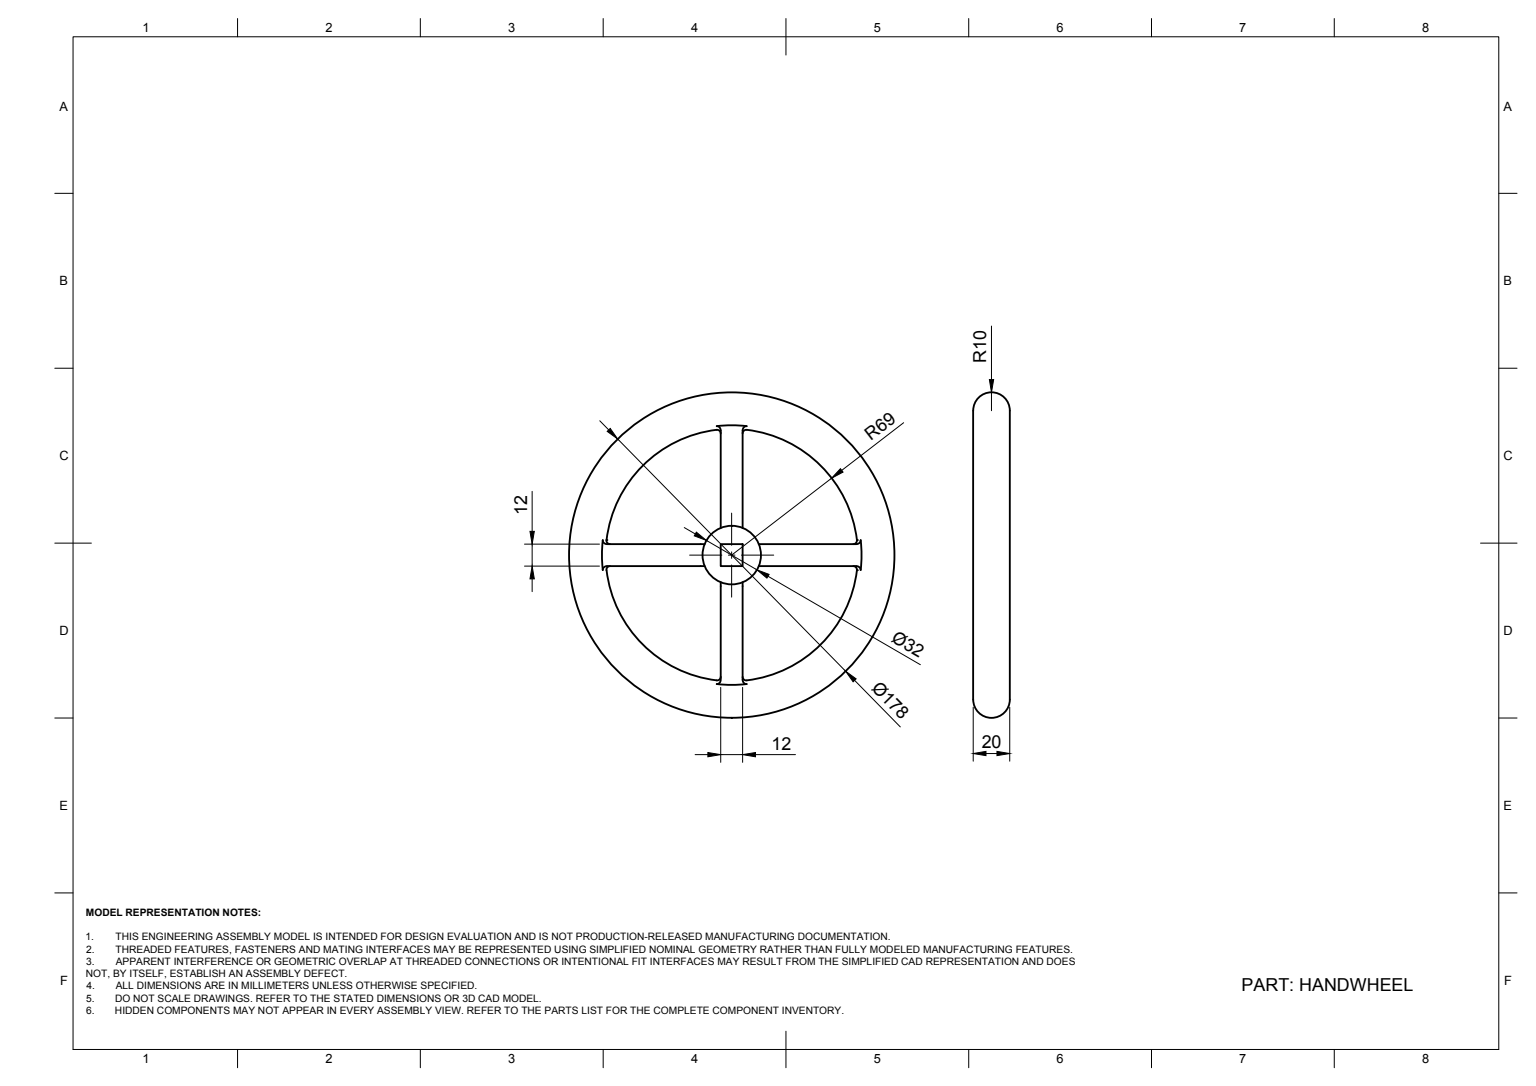
ISO-10303-21;
HEADER;
/* Generated by software containing ST-Developer
 * from STEP Tools, Inc. (www.steptools.com) 
 */

FILE_DESCRIPTION(
/* description */ (''),
/* implementation_level */ '2;1');

FILE_NAME(
/* name */ 'HANDWHEEL.step',
/* time_stamp */ '2026-10-04T02:10:06-07:00',
/* author */ (''),
/* organization */ (''),
/* preprocessor_version */ 'ST-DEVELOPER v20.2',
/* originating_system */ 'Autodesk Translation Framework v15.15.0.0',
/* authorisation */ '');

FILE_SCHEMA (('AUTOMOTIVE_DESIGN { 1 0 10303 214 3 1 1 }'));
ENDSEC;

DATA;
#10=MECHANICAL_DESIGN_GEOMETRIC_PRESENTATION_REPRESENTATION('',(#149),#9668);
#67=(
BOUNDED_SURFACE()
B_SPLINE_SURFACE(3,2,((#8974,#8975,#8976),(#8977,#8978,#8979),(#8980,#8981,
#8982),(#8983,#8984,#8985),(#8986,#8987,#8988),(#8989,#8990,#8991),(#8992,
#8993,#8994),(#8995,#8996,#8997),(#8998,#8999,#9000),(#9001,#9002,#9003),
(#9004,#9005,#9006),(#9007,#9008,#9009),(#9010,#9011,#9012),(#9013,#9014,
#9015),(#9016,#9017,#9018),(#9019,#9020,#9021),(#9022,#9023,#9024),(#9025,
#9026,#9027)),.UNSPECIFIED.,.F.,.F.,.F.)
B_SPLINE_SURFACE_WITH_KNOTS((4,1,1,1,1,1,1,1,1,1,1,1,1,1,1,4),(3,3),(0.0314788030428868,
0.0324522874563819,0.0334257718698771,0.0353727406968673,0.0363462251103625,
0.0373197095238576,0.0382931939373528,0.0392666783508479,0.0402401627643431,
0.0412136471778382,0.0421871315913334,0.0431606160048285,0.0441341004183236,
0.0451075848318188,0.0460810692453139,0.0470545536588091),(0.,1.),
 .UNSPECIFIED.)
GEOMETRIC_REPRESENTATION_ITEM()
RATIONAL_B_SPLINE_SURFACE(((1.,0.673965297618148,1.),(1.,0.673166296515258,
1.),(1.,0.671622878424884,1.),(1.,0.668872043360916,1.),(1.,0.6666737415125,
1.),(1.,0.665066367000124,1.),(1.,0.664191179384959,1.),(1.,0.663664801981856,
1.),(1.,0.663490402453091,1.),(1.,0.663673371681184,1.),(1.,0.664201607885415,
1.),(1.,0.66506767873011,1.),(1.,0.666279408316226,1.),(1.,0.667792932640577,
1.),(1.,0.669583017900756,1.),(1.,0.671633975311695,1.),(1.,0.673174922786531,
1.),(1.,0.673980190168732,1.)))
REPRESENTATION_ITEM('')
SURFACE()
);
#68=(
BOUNDED_SURFACE()
B_SPLINE_SURFACE(3,2,((#9028,#9029,#9030),(#9031,#9032,#9033),(#9034,#9035,
#9036),(#9037,#9038,#9039),(#9040,#9041,#9042),(#9043,#9044,#9045),(#9046,
#9047,#9048),(#9049,#9050,#9051),(#9052,#9053,#9054),(#9055,#9056,#9057),
(#9058,#9059,#9060),(#9061,#9062,#9063),(#9064,#9065,#9066),(#9067,#9068,
#9069),(#9070,#9071,#9072),(#9073,#9074,#9075),(#9076,#9077,#9078),(#9079,
#9080,#9081)),.UNSPECIFIED.,.F.,.F.,.F.)
B_SPLINE_SURFACE_WITH_KNOTS((4,1,1,1,1,1,1,1,1,1,1,1,1,1,1,4),(3,3),(0.0306904631349172,
0.0316643361466102,0.0326382091583032,0.0336120821699963,0.0345859551816893,
0.0355598281933823,0.0365337012050753,0.0375075742167683,0.0384814472284614,
0.0394553202401544,0.0404291932518474,0.0414030662635404,0.0423769392752334,
0.0433508122869265,0.0443246852986195,0.0462724313220055),(0.,1.),
 .UNSPECIFIED.)
GEOMETRIC_REPRESENTATION_ITEM()
RATIONAL_B_SPLINE_SURFACE(((1.,0.673964349039136,1.),(1.,0.673168502978567,
1.),(1.,0.671643925861953,1.),(1.,0.669562296886318,1.),(1.,0.667767007356651,
1.),(1.,0.666266776870979,1.),(1.,0.665071978074277,1.),(1.,0.664194007330874,
1.),(1.,0.663665542131989,1.),(1.,0.663490103902602,1.),(1.,0.663673710164509,
1.),(1.,0.664205908065376,1.),(1.,0.665074561266886,1.),(1.,0.666270920547672,
1.),(1.,0.667799410011383,1.),(1.,0.670197938500333,1.),(1.,0.672375755500364,
1.),(1.,0.673978916833767,1.)))
REPRESENTATION_ITEM('')
SURFACE()
);
#69=(
BOUNDED_SURFACE()
B_SPLINE_SURFACE(3,2,((#9082,#9083,#9084),(#9085,#9086,#9087),(#9088,#9089,
#9090),(#9091,#9092,#9093),(#9094,#9095,#9096),(#9097,#9098,#9099),(#9100,
#9101,#9102),(#9103,#9104,#9105),(#9106,#9107,#9108),(#9109,#9110,#9111),
(#9112,#9113,#9114),(#9115,#9116,#9117),(#9118,#9119,#9120),(#9121,#9122,
#9123),(#9124,#9125,#9126),(#9127,#9128,#9129),(#9130,#9131,#9132),(#9133,
#9134,#9135)),.UNSPECIFIED.,.F.,.F.,.F.)
B_SPLINE_SURFACE_WITH_KNOTS((4,1,1,1,1,1,1,1,1,1,1,1,1,1,1,4),(3,3),(0.0305897871911959,
0.0315636944986189,0.0325376018060419,0.0335115091134649,0.0344854164208879,
0.0354593237283109,0.0364332310357338,0.0374071383431568,0.0383810456505798,
0.0393549529580028,0.0403288602654258,0.0413027675728487,0.0422766748802717,
0.0432505821876947,0.0442244894951177,0.0461723041099637),(0.,1.),
 .UNSPECIFIED.)
GEOMETRIC_REPRESENTATION_ITEM()
RATIONAL_B_SPLINE_SURFACE(((1.,0.673964296834234,1.),(1.,0.673168609933157,
1.),(1.,0.671645019887839,1.),(1.,0.669565127304379,1.),(1.,0.667766560497273,
1.),(1.,0.666266474426915,1.),(1.,0.66507215658795,1.),(1.,0.664195156886529,
1.),(1.,0.663665573830476,1.),(1.,0.663490167959275,1.),(1.,0.663673406028792,
1.),(1.,0.664206149646574,1.),(1.,0.665075135400244,1.),(1.,0.666270395103817,
1.),(1.,0.667798233506142,1.),(1.,0.670199686629813,1.),(1.,0.672377030394903,
1.),(1.,0.673978715902987,1.)))
REPRESENTATION_ITEM('')
SURFACE()
);
#70=(
BOUNDED_SURFACE()
B_SPLINE_SURFACE(3,2,((#9136,#9137,#9138),(#9139,#9140,#9141),(#9142,#9143,
#9144),(#9145,#9146,#9147),(#9148,#9149,#9150),(#9151,#9152,#9153),(#9154,
#9155,#9156),(#9157,#9158,#9159),(#9160,#9161,#9162),(#9163,#9164,#9165),
(#9166,#9167,#9168),(#9169,#9170,#9171),(#9172,#9173,#9174),(#9175,#9176,
#9177),(#9178,#9179,#9180),(#9181,#9182,#9183),(#9184,#9185,#9186),(#9187,
#9188,#9189)),.UNSPECIFIED.,.F.,.F.,.F.)
B_SPLINE_SURFACE_WITH_KNOTS((4,1,1,1,1,1,1,1,1,1,1,1,1,1,1,4),(3,3),(0.0315789108977846,
0.0325523529389518,0.0335257949801189,0.0354726790624532,0.0364461211036204,
0.0374195631447876,0.0383930051859547,0.0393664472271219,0.040339889268289,
0.0413133313094562,0.0422867733506233,0.0432602153917905,0.0442336574329576,
0.0452070994741248,0.046180541515292,0.0471539835564591),(0.,1.),
 .UNSPECIFIED.)
GEOMETRIC_REPRESENTATION_ITEM()
RATIONAL_B_SPLINE_SURFACE(((1.,0.673965492863365,1.),(1.,0.673165826863236,
1.),(1.,0.671620469526443,1.),(1.,0.668874652098692,1.),(1.,0.666674941728974,
1.),(1.,0.665065162761098,1.),(1.,0.664191461531519,1.),(1.,0.663664604196809,
1.),(1.,0.663490522562251,1.),(1.,0.663673087023803,1.),(1.,0.664200791428412,
1.),(1.,0.665067176842279,1.),(1.,0.666279817333014,1.),(1.,0.667791010794828,
1.),(1.,0.669580698382089,1.),(1.,0.671631849583161,1.),(1.,0.673175667819509,
1.),(1.,0.673979886421463,1.)))
REPRESENTATION_ITEM('')
SURFACE()
);
#71=(
BOUNDED_SURFACE()
B_SPLINE_SURFACE(3,2,((#9190,#9191,#9192),(#9193,#9194,#9195),(#9196,#9197,
#9198),(#9199,#9200,#9201),(#9202,#9203,#9204),(#9205,#9206,#9207),(#9208,
#9209,#9210),(#9211,#9212,#9213),(#9214,#9215,#9216),(#9217,#9218,#9219),
(#9220,#9221,#9222),(#9223,#9224,#9225),(#9226,#9227,#9228),(#9229,#9230,
#9231),(#9232,#9233,#9234),(#9235,#9236,#9237)),.UNSPECIFIED.,.F.,.F.,.F.)
B_SPLINE_SURFACE_WITH_KNOTS((4,1,1,1,1,1,1,1,1,1,1,1,1,4),(3,3),(0.03215789731342,
0.0331313751868945,0.034104853060369,0.0350783309338435,0.0360518088073179,
0.0370252866807924,0.0379987645542669,0.0389722424277414,0.0399457203012159,
0.0418926760481649,0.0438396317951138,0.0457865875420628,0.0467600654155373,
0.0477335432890118),(-8.08454907084105E-6,1.),.UNSPECIFIED.)
GEOMETRIC_REPRESENTATION_ITEM()
RATIONAL_B_SPLINE_SURFACE(((1.00000527170182,0.673964387359616,1.),(1.00000528471687,
0.673159453411099,1.),(1.00000530961685,0.671619480347489,1.),(1.00000534275063,
0.669570276226346,1.),(1.00000537166522,0.66778201413489,1.),(1.00000539609675,
0.666271012581043,1.),(1.00000541568478,0.665059564372101,1.),(1.00000542974255,
0.664190142086893,1.),(1.000005438313,0.663660090710924,1.),(1.00000544199604,
0.663432308407853,1.),(1.00000543253772,0.664017270646154,1.),(1.00000539844928,
0.666125517336438,1.),(1.00000535391695,0.668879680311451,1.),(1.00000530941503,
0.671631962440139,1.),(1.00000528444356,0.673176357213759,1.),(1.00000527151599,
0.673975880021096,1.)))
REPRESENTATION_ITEM('')
SURFACE()
);
#72=(
BOUNDED_SURFACE()
B_SPLINE_SURFACE(3,2,((#9238,#9239,#9240),(#9241,#9242,#9243),(#9244,#9245,
#9246),(#9247,#9248,#9249),(#9250,#9251,#9252),(#9253,#9254,#9255),(#9256,
#9257,#9258),(#9259,#9260,#9261),(#9262,#9263,#9264),(#9265,#9266,#9267),
(#9268,#9269,#9270),(#9271,#9272,#9273),(#9274,#9275,#9276),(#9277,#9278,
#9279),(#9280,#9281,#9282),(#9283,#9284,#9285)),.UNSPECIFIED.,.F.,.F.,.F.)
B_SPLINE_SURFACE_WITH_KNOTS((4,1,1,1,1,1,1,1,1,1,1,1,1,4),(3,3),(0.0300049518513901,
0.031953018177045,0.0329270513398724,0.0339010845026998,0.0348751176655272,
0.0358491508283546,0.036823183991182,0.0377972171540094,0.0387712503168368,
0.0397452834796642,0.041693349805319,0.0426673829681464,0.0436414161309738,
0.0455894824566286),(0.,1.),.UNSPECIFIED.)
GEOMETRIC_REPRESENTATION_ITEM()
RATIONAL_B_SPLINE_SURFACE(((1.,0.673964297815332,1.),(1.,0.672372618458235,
1.),(1.,0.670191181394266,1.),(1.,0.667767841290405,1.),(1.,0.666265347639804,
1.),(1.,0.665072121147338,1.),(1.,0.664201207028703,1.),(1.,0.663666605647771,
1.),(1.,0.663490715236844,1.),(1.,0.663670119784287,1.),(1.,0.664385152559804,
1.),(1.,0.665767066134064,1.),(1.,0.66778345083312,1.),(1.,0.670206332337341,
1.),(1.,0.672382580991143,1.),(1.,0.673977852527306,1.)))
REPRESENTATION_ITEM('')
SURFACE()
);
#73=(
BOUNDED_SURFACE()
B_SPLINE_SURFACE(3,2,((#9286,#9287,#9288),(#9289,#9290,#9291),(#9292,#9293,
#9294),(#9295,#9296,#9297),(#9298,#9299,#9300),(#9301,#9302,#9303),(#9304,
#9305,#9306),(#9307,#9308,#9309),(#9310,#9311,#9312),(#9313,#9314,#9315),
(#9316,#9317,#9318),(#9319,#9320,#9321),(#9322,#9323,#9324),(#9325,#9326,
#9327),(#9328,#9329,#9330),(#9331,#9332,#9333),(#9334,#9335,#9336),(#9337,
#9338,#9339),(#9340,#9341,#9342)),.UNSPECIFIED.,.F.,.F.,.F.)
B_SPLINE_SURFACE_WITH_KNOTS((4,1,1,1,1,1,1,1,1,1,1,1,1,1,1,1,4),(3,3),(0.0317649381765832,
0.0327383392942574,0.0337117404119316,0.0346851415296058,0.03565854264728,
0.0366319437649542,0.0376053448826284,0.0385787460003026,0.0395521471179768,
0.040525548235651,0.0414989493533253,0.0424723504709995,0.0434457515886737,
0.0444191527063479,0.0453925538240221,0.0463659549416963,0.0473393560593705),
(0.,1.),.UNSPECIFIED.)
GEOMETRIC_REPRESENTATION_ITEM()
RATIONAL_B_SPLINE_SURFACE(((1.,0.673965909365134,1.),(1.,0.673164818236142,
1.),(1.,0.671618061862569,1.),(1.,0.669564320284071,1.),(1.,0.66777759511695,
1.),(1.,0.666273471258361,1.),(1.,0.665063410818969,1.),(1.,0.664191967652661,
1.),(1.,0.663664156821065,1.),(1.,0.663490769293391,1.),(1.,0.663672536496092,
1.),(1.,0.664199292987571,1.),(1.,0.665067031441957,1.),(1.,0.666280071948857,
1.),(1.,0.66778774864528,1.),(1.,0.669576760671401,1.),(1.,0.671629936935393,
1.),(1.,0.673176919539912,1.),(1.,0.673979374441674,1.)))
REPRESENTATION_ITEM('')
SURFACE()
);
#74=(
BOUNDED_SURFACE()
B_SPLINE_SURFACE(3,2,((#9343,#9344,#9345),(#9346,#9347,#9348),(#9349,#9350,
#9351),(#9352,#9353,#9354),(#9355,#9356,#9357),(#9358,#9359,#9360),(#9361,
#9362,#9363),(#9364,#9365,#9366),(#9367,#9368,#9369),(#9370,#9371,#9372),
(#9373,#9374,#9375),(#9376,#9377,#9378),(#9379,#9380,#9381),(#9382,#9383,
#9384),(#9385,#9386,#9387),(#9388,#9389,#9390),(#9391,#9392,#9393)),
 .UNSPECIFIED.,.F.,.F.,.F.)
B_SPLINE_SURFACE_WITH_KNOTS((4,1,1,1,1,1,1,1,1,1,1,1,1,1,4),(3,3),(0.0304023584176636,
0.0313763197495467,0.0323502810814299,0.0333242424133131,0.0342982037451962,
0.0352721650770794,0.0362461264089626,0.0372200877408457,0.0381940490727289,
0.0391680104046121,0.0401419717364953,0.0420898944002616,0.0430638557321448,
0.0440378170640279,0.0459857397277943),(0.,1.),.UNSPECIFIED.)
GEOMETRIC_REPRESENTATION_ITEM()
RATIONAL_B_SPLINE_SURFACE(((1.,0.673964240667089,1.),(1.,0.673168704865034,
1.),(1.,0.671646043506943,1.),(1.,0.669571927360062,1.),(1.,0.667765968900773,
1.),(1.,0.666266091842261,1.),(1.,0.665072243840693,1.),(1.,0.664197515743925,
1.),(1.,0.663665655019745,1.),(1.,0.663490373557035,1.),(1.,0.663672476132646,
1.),(1.,0.664385168150455,1.),(1.,0.665762507320331,1.),(1.,0.667794613454947,
1.),(1.,0.670202685638588,1.),(1.,0.672379152055614,1.),(1.,0.6739783830491,
1.)))
REPRESENTATION_ITEM('')
SURFACE()
);
#127=SHAPE_REPRESENTATION_RELATIONSHIP('SRR','None',#9720,#138);
#138=ADVANCED_BREP_SHAPE_REPRESENTATION('',(#160),#9665);
#149=STYLED_ITEM('',(#9775),#160);
#160=MANIFOLD_SOLID_BREP('Body1',#3889);
#260=FACE_BOUND('',#1262,.T.);
#261=FACE_BOUND('',#1263,.T.);
#262=FACE_BOUND('',#1264,.T.);
#263=FACE_BOUND('',#1266,.T.);
#264=FACE_BOUND('',#1268,.T.);
#332=PLANE('',#4327);
#333=PLANE('',#4328);
#334=PLANE('',#4329);
#335=PLANE('',#4332);
#336=PLANE('',#4336);
#337=PLANE('',#4339);
#338=PLANE('',#4343);
#339=PLANE('',#4346);
#340=PLANE('',#4349);
#341=PLANE('',#4350);
#342=PLANE('',#4351);
#343=PLANE('',#4352);
#344=PLANE('',#4353);
#345=PLANE('',#4354);
#346=PLANE('',#4363);
#347=PLANE('',#4365);
#348=PLANE('',#4380);
#349=PLANE('',#4381);
#350=PLANE('',#4382);
#351=PLANE('',#4383);
#352=PLANE('',#4384);
#353=PLANE('',#4385);
#504=LINE('',#7172,#695);
#505=LINE('',#7263,#696);
#506=LINE('',#7276,#697);
#507=LINE('',#7290,#698);
#508=LINE('',#7384,#699);
#509=LINE('',#7397,#700);
#510=LINE('',#7440,#701);
#511=LINE('',#7444,#702);
#512=LINE('',#7477,#703);
#513=LINE('',#7481,#704);
#514=LINE('',#7512,#705);
#515=LINE('',#7516,#706);
#516=LINE('',#7578,#707);
#517=LINE('',#7582,#708);
#518=LINE('',#7701,#709);
#519=LINE('',#7714,#710);
#520=LINE('',#7728,#711);
#521=LINE('',#7823,#712);
#522=LINE('',#7932,#713);
#523=LINE('',#8044,#714);
#524=LINE('',#8149,#715);
#525=LINE('',#8162,#716);
#526=LINE('',#8176,#717);
#527=LINE('',#8274,#718);
#528=LINE('',#8925,#719);
#529=LINE('',#8930,#720);
#530=LINE('',#8943,#721);
#531=LINE('',#8945,#722);
#532=LINE('',#8947,#723);
#533=LINE('',#8948,#724);
#534=LINE('',#8952,#725);
#535=LINE('',#8954,#726);
#536=LINE('',#8956,#727);
#537=LINE('',#8957,#728);
#538=LINE('',#8959,#729);
#539=LINE('',#8960,#730);
#540=LINE('',#8962,#731);
#541=LINE('',#8964,#732);
#695=VECTOR('',#5230,51.1691161062453);
#696=VECTOR('',#5231,51.1691161062453);
#697=VECTOR('',#5232,16.);
#698=VECTOR('',#5235,51.1691161062453);
#699=VECTOR('',#5236,51.1691161062453);
#700=VECTOR('',#5237,16.);
#701=VECTOR('',#5246,51.1691161062453);
#702=VECTOR('',#5249,51.1691161062452);
#703=VECTOR('',#5256,51.1691161062453);
#704=VECTOR('',#5259,51.1691161062453);
#705=VECTOR('',#5264,51.1691161062453);
#706=VECTOR('',#5267,51.1691161062453);
#707=VECTOR('',#5280,51.1691161062453);
#708=VECTOR('',#5283,51.1691161062453);
#709=VECTOR('',#5288,51.1691161062453);
#710=VECTOR('',#5289,16.);
#711=VECTOR('',#5292,51.1691161062453);
#712=VECTOR('',#5293,16.);
#713=VECTOR('',#5296,16.);
#714=VECTOR('',#5299,16.);
#715=VECTOR('',#5302,51.1691161062453);
#716=VECTOR('',#5303,16.);
#717=VECTOR('',#5306,51.1691161062453);
#718=VECTOR('',#5307,16.);
#719=VECTOR('',#5336,16.);
#720=VECTOR('',#5341,16.);
#721=VECTOR('',#5362,12.);
#722=VECTOR('',#5363,12.);
#723=VECTOR('',#5364,12.);
#724=VECTOR('',#5365,12.);
#725=VECTOR('',#5368,12.);
#726=VECTOR('',#5369,12.);
#727=VECTOR('',#5370,12.);
#728=VECTOR('',#5371,12.);
#729=VECTOR('',#5374,20.);
#730=VECTOR('',#5375,20.);
#731=VECTOR('',#5378,20.);
#732=VECTOR('',#5381,20.);
#807=CYLINDRICAL_SURFACE('',#4367,16.);
#956=FACE_OUTER_BOUND('',#1244,.T.);
#957=FACE_OUTER_BOUND('',#1245,.T.);
#958=FACE_OUTER_BOUND('',#1246,.T.);
#959=FACE_OUTER_BOUND('',#1247,.T.);
#960=FACE_OUTER_BOUND('',#1248,.T.);
#961=FACE_OUTER_BOUND('',#1249,.T.);
#962=FACE_OUTER_BOUND('',#1250,.T.);
#963=FACE_OUTER_BOUND('',#1251,.T.);
#964=FACE_OUTER_BOUND('',#1252,.T.);
#965=FACE_OUTER_BOUND('',#1253,.T.);
#966=FACE_OUTER_BOUND('',#1254,.T.);
#967=FACE_OUTER_BOUND('',#1255,.T.);
#968=FACE_OUTER_BOUND('',#1256,.T.);
#969=FACE_OUTER_BOUND('',#1257,.T.);
#970=FACE_OUTER_BOUND('',#1258,.T.);
#971=FACE_OUTER_BOUND('',#1259,.T.);
#972=FACE_OUTER_BOUND('',#1260,.T.);
#973=FACE_OUTER_BOUND('',#1261,.T.);
#974=FACE_OUTER_BOUND('',#1265,.T.);
#975=FACE_OUTER_BOUND('',#1267,.T.);
#976=FACE_OUTER_BOUND('',#1269,.T.);
#977=FACE_OUTER_BOUND('',#1270,.T.);
#978=FACE_OUTER_BOUND('',#1271,.T.);
#979=FACE_OUTER_BOUND('',#1272,.T.);
#980=FACE_OUTER_BOUND('',#1273,.T.);
#981=FACE_OUTER_BOUND('',#1274,.T.);
#982=FACE_OUTER_BOUND('',#1275,.T.);
#983=FACE_OUTER_BOUND('',#1276,.T.);
#984=FACE_OUTER_BOUND('',#1277,.T.);
#985=FACE_OUTER_BOUND('',#1278,.T.);
#986=FACE_OUTER_BOUND('',#1279,.T.);
#987=FACE_OUTER_BOUND('',#1280,.T.);
#988=FACE_OUTER_BOUND('',#1281,.T.);
#989=FACE_OUTER_BOUND('',#1282,.T.);
#990=FACE_OUTER_BOUND('',#1283,.T.);
#991=FACE_OUTER_BOUND('',#1284,.T.);
#992=FACE_OUTER_BOUND('',#1285,.T.);
#993=FACE_OUTER_BOUND('',#1286,.T.);
#994=FACE_OUTER_BOUND('',#1287,.T.);
#995=FACE_OUTER_BOUND('',#1288,.T.);
#1244=EDGE_LOOP('',(#3221,#3222,#3223,#3224,#3225,#3226));
#1245=EDGE_LOOP('',(#3227,#3228,#3229,#3230,#3231,#3232));
#1246=EDGE_LOOP('',(#3233,#3234,#3235,#3236,#3237,#3238));
#1247=EDGE_LOOP('',(#3239,#3240,#3241,#3242,#3243,#3244,#3245));
#1248=EDGE_LOOP('',(#3246,#3247,#3248,#3249,#3250,#3251));
#1249=EDGE_LOOP('',(#3252,#3253,#3254,#3255,#3256,#3257,#3258));
#1250=EDGE_LOOP('',(#3259,#3260,#3261,#3262,#3263,#3264));
#1251=EDGE_LOOP('',(#3265,#3266,#3267,#3268,#3269,#3270));
#1252=EDGE_LOOP('',(#3271,#3272,#3273,#3274,#3275,#3276));
#1253=EDGE_LOOP('',(#3277,#3278,#3279,#3280,#3281,#3282));
#1254=EDGE_LOOP('',(#3283,#3284,#3285,#3286,#3287,#3288));
#1255=EDGE_LOOP('',(#3289,#3290,#3291,#3292,#3293,#3294));
#1256=EDGE_LOOP('',(#3295,#3296,#3297,#3298,#3299,#3300));
#1257=EDGE_LOOP('',(#3301,#3302,#3303,#3304,#3305,#3306));
#1258=EDGE_LOOP('',(#3307,#3308,#3309,#3310,#3311,#3312,#3313,#3314,#3315,
#3316,#3317,#3318,#3319,#3320,#3321,#3322,#3323,#3324,#3325,#3326,#3327,
#3328,#3329,#3330,#3331,#3332,#3333,#3334,#3335,#3336,#3337,#3338,#3339,
#3340,#3341,#3342));
#1259=EDGE_LOOP('',(#3343,#3344,#3345,#3346,#3347,#3348));
#1260=EDGE_LOOP('',(#3349,#3350,#3351,#3352,#3353,#3354));
#1261=EDGE_LOOP('',(#3355,#3356,#3357,#3358,#3359,#3360,#3361,#3362,#3363,
#3364,#3365,#3366));
#1262=EDGE_LOOP('',(#3367,#3368,#3369,#3370));
#1263=EDGE_LOOP('',(#3371,#3372,#3373,#3374));
#1264=EDGE_LOOP('',(#3375,#3376,#3377,#3378));
#1265=EDGE_LOOP('',(#3379));
#1266=EDGE_LOOP('',(#3380,#3381,#3382,#3383));
#1267=EDGE_LOOP('',(#3384));
#1268=EDGE_LOOP('',(#3385,#3386,#3387,#3388));
#1269=EDGE_LOOP('',(#3389,#3390,#3391,#3392));
#1270=EDGE_LOOP('',(#3393,#3394,#3395,#3396));
#1271=EDGE_LOOP('',(#3397,#3398,#3399,#3400));
#1272=EDGE_LOOP('',(#3401,#3402,#3403,#3404));
#1273=EDGE_LOOP('',(#3405,#3406,#3407,#3408,#3409));
#1274=EDGE_LOOP('',(#3410,#3411,#3412,#3413));
#1275=EDGE_LOOP('',(#3414,#3415,#3416,#3417,#3418));
#1276=EDGE_LOOP('',(#3419,#3420,#3421,#3422));
#1277=EDGE_LOOP('',(#3423,#3424,#3425,#3426));
#1278=EDGE_LOOP('',(#3427,#3428,#3429,#3430));
#1279=EDGE_LOOP('',(#3431,#3432,#3433,#3434));
#1280=EDGE_LOOP('',(#3435,#3436,#3437,#3438));
#1281=EDGE_LOOP('',(#3439,#3440,#3441,#3442,#3443));
#1282=EDGE_LOOP('',(#3444,#3445,#3446,#3447,#3448));
#1283=EDGE_LOOP('',(#3449,#3450,#3451,#3452,#3453));
#1284=EDGE_LOOP('',(#3454,#3455,#3456,#3457,#3458));
#1285=EDGE_LOOP('',(#3459,#3460,#3461,#3462,#3463));
#1286=EDGE_LOOP('',(#3464,#3465,#3466,#3467,#3468));
#1287=EDGE_LOOP('',(#3469,#3470,#3471,#3472,#3473));
#1288=EDGE_LOOP('',(#3474,#3475,#3476,#3477,#3478));
#1371=B_SPLINE_CURVE_WITH_KNOTS('',3,(#7174,#7175,#7176,#7177,#7178,#7179,
#7180,#7181,#7182,#7183,#7184,#7185,#7186,#7187,#7188,#7189,#7190,#7191,
#7192,#7193,#7194,#7195,#7196,#7197,#7198,#7199,#7200,#7201,#7202,#7203,
#7204,#7205,#7206,#7207,#7208,#7209,#7210,#7211,#7212,#7213,#7214,#7215,
#7216,#7217,#7218,#7219,#7220,#7221,#7222,#7223,#7224,#7225,#7226,#7227,
#7228,#7229,#7230,#7231,#7232,#7233,#7234,#7235,#7236,#7237,#7238,#7239,
#7240,#7241,#7242,#7243,#7244,#7245,#7246,#7247,#7248,#7249,#7250,#7251,
#7252,#7253,#7254,#7255,#7256,#7257,#7258,#7259,#7260,#7261),
 .UNSPECIFIED.,.F.,.F.,(4,3,3,3,3,3,3,3,3,3,3,3,3,3,3,3,3,3,3,3,3,3,3,3,
3,3,3,3,3,4),(0.,0.000406240529099286,0.00137938545876311,0.00157223368396575,
0.00235712040686395,0.00235835052594862,0.0031444673679315,0.00333814638883581,
0.00417473181206057,0.00431968916279243,0.00471670105189724,0.00530146021537391,
0.00628278928089295,0.00628893473586299,0.00698096938738472,0.00707505157784587,
0.00726415374654744,0.00786116841982874,0.00824590532689442,0.00864728526181162,
0.00916646995968722,0.00922701267009175,0.00943340210379449,0.0101214219001075,
0.0102072274047249,0.0108935730580786,0.0110056357877602,0.0120607068335696,
0.0121610933723902,0.012577869471726),.UNSPECIFIED.);
#1372=B_SPLINE_CURVE_WITH_KNOTS('',3,(#7265,#7266,#7267,#7268,#7269,#7270,
#7271,#7272,#7273,#7274),.UNSPECIFIED.,.F.,.F.,(4,2,2,2,4),(-0.917009726243287,
-0.836713680249397,-0.758350426571219,-0.683089589535854,-0.610699399852799),
 .UNSPECIFIED.);
#1373=B_SPLINE_CURVE_WITH_KNOTS('',3,(#7277,#7278,#7279,#7280,#7281,#7282,
#7283,#7284,#7285,#7286),.UNSPECIFIED.,.F.,.F.,(4,2,2,2,4),(-0.610699399852799,
-0.538309210169743,-0.463048373134379,-0.384685119456201,-0.30438907346231),
 .UNSPECIFIED.);
#1374=B_SPLINE_CURVE_WITH_KNOTS('',3,(#7292,#7293,#7294,#7295,#7296,#7297,
#7298,#7299,#7300,#7301,#7302,#7303,#7304,#7305,#7306,#7307,#7308,#7309,
#7310,#7311,#7312,#7313,#7314,#7315,#7316,#7317,#7318,#7319,#7320,#7321,
#7322,#7323,#7324,#7325,#7326,#7327,#7328,#7329,#7330,#7331,#7332,#7333,
#7334,#7335,#7336,#7337,#7338,#7339,#7340,#7341,#7342,#7343,#7344,#7345,
#7346,#7347,#7348,#7349,#7350,#7351,#7352,#7353,#7354,#7355,#7356,#7357,
#7358,#7359,#7360,#7361,#7362,#7363,#7364,#7365,#7366,#7367,#7368,#7369,
#7370,#7371,#7372,#7373,#7374,#7375,#7376,#7377,#7378,#7379,#7380,#7381,
#7382),.UNSPECIFIED.,.F.,.F.,(4,3,3,3,3,3,3,3,3,3,3,3,3,3,3,3,3,3,3,3,3,
3,3,3,3,3,3,3,3,3,4),(2.60208521396521E-18,0.000400192674595473,0.00127218628897403,
0.00137785726958694,0.00157876092999531,0.00227142090955615,0.0023618191099302,
0.00236814139499296,0.00315752185999062,0.00334675544179567,0.0043315650279144,
0.00473628278998593,0.00531664189634561,0.00552566325498358,0.0061211332819969,
0.00630145520527624,0.00631504371998124,0.00698165466480908,0.00728672101907334,
0.00789380464997654,0.00827095042480516,0.0086831851149742,0.00918475578885096,
0.00925631171880029,0.00947256557997185,0.0102418473576122,0.0110513265099672,
0.0112276216640443,0.0118264377408911,0.0122140928457701,0.0126300874399625),
 .UNSPECIFIED.);
#1375=B_SPLINE_CURVE_WITH_KNOTS('',3,(#7386,#7387,#7388,#7389,#7390,#7391,
#7392,#7393,#7394,#7395),.UNSPECIFIED.,.F.,.F.,(4,2,2,2,4),(0.30438907346231,
0.384685119456201,0.463048373134379,0.538309210169743,0.610699399852799),
 .UNSPECIFIED.);
#1376=B_SPLINE_CURVE_WITH_KNOTS('',3,(#7398,#7399,#7400,#7401,#7402,#7403,
#7404,#7405,#7406,#7407),.UNSPECIFIED.,.F.,.F.,(4,2,2,2,4),(0.610699399852799,
0.683089589535854,0.758350426571219,0.836713680249397,0.917009726243287),
 .UNSPECIFIED.);
#1377=B_SPLINE_CURVE_WITH_KNOTS('',3,(#7411,#7412,#7413,#7414,#7415,#7416,
#7417,#7418,#7419,#7420,#7421,#7422),.UNSPECIFIED.,.F.,.F.,(4,2,2,2,2,4),
(-0.362882917350416,-0.274135453989767,-0.182717407796491,-0.100687086335371,
-0.0480780172014038,0.),.UNSPECIFIED.);
#1378=B_SPLINE_CURVE_WITH_KNOTS('',3,(#7425,#7426,#7427,#7428,#7429,#7430,
#7431,#7432,#7433,#7434,#7435,#7436),.UNSPECIFIED.,.F.,.F.,(4,2,2,2,2,4),
(-0.365096706754078,-0.31691860503495,-0.264216176140628,-0.181784514384503,
-0.0898745758923246,-9.99999994033989E-7),.UNSPECIFIED.);
#1379=B_SPLINE_CURVE_WITH_KNOTS('',3,(#7446,#7447,#7448,#7449,#7450,#7451,
#7452,#7453,#7454,#7455,#7456,#7457),.UNSPECIFIED.,.F.,.F.,(4,2,2,2,2,4),
(-0.362876736231209,-0.274133802851703,-0.182716474898388,-0.100684866470481,
-0.0480764814879336,0.),.UNSPECIFIED.);
#1380=B_SPLINE_CURVE_WITH_KNOTS('',3,(#7462,#7463,#7464,#7465,#7466,#7467,
#7468,#7469,#7470,#7471,#7472,#7473),.UNSPECIFIED.,.F.,.F.,(4,2,2,2,2,4),
(-0.365091922937845,-0.316913549080402,-0.26421121051335,-0.181781618094101,
-0.089862766267777,-9.99999992201683E-7),.UNSPECIFIED.);
#1381=B_SPLINE_CURVE_WITH_KNOTS('',3,(#7483,#7484,#7485,#7486,#7487,#7488,
#7489,#7490,#7491,#7492,#7493,#7494),.UNSPECIFIED.,.F.,.F.,(4,2,2,2,2,4),
(-0.362882338171715,-0.274127578782018,-0.182717811491084,-0.100689968817147,
-0.0480792415446598,0.),.UNSPECIFIED.);
#1382=B_SPLINE_CURVE_WITH_KNOTS('',3,(#7497,#7498,#7499,#7500,#7501,#7502,
#7503,#7504,#7505,#7506,#7507,#7508),.UNSPECIFIED.,.F.,.F.,(4,2,2,2,2,4),
(-0.365095174259356,-0.316917006202739,-0.264214779903918,-0.181783926909875,
-0.0898710353312815,-9.99999992257194E-7),.UNSPECIFIED.);
#1383=B_SPLINE_CURVE_WITH_KNOTS('',3,(#7518,#7519,#7520,#7521,#7522,#7523,
#7524,#7525,#7526,#7527,#7528,#7529),.UNSPECIFIED.,.F.,.F.,(4,2,2,2,2,4),
(-0.362869289557713,-0.274152784534485,-0.182713567211171,-0.100681309588015,
-0.0480754657457727,-6.35607511623171E-8),.UNSPECIFIED.);
#1384=B_SPLINE_CURVE_WITH_KNOTS('',3,(#7534,#7535,#7536,#7537,#7538,#7539,
#7540,#7541,#7542,#7543,#7544,#7545),.UNSPECIFIED.,.F.,.F.,(4,2,2,2,2,4),
(-0.365071317763414,-0.316894297426638,-0.264193403878945,-0.181773042602845,
-0.0898848198288387,0.),.UNSPECIFIED.);
#1385=B_SPLINE_CURVE_WITH_KNOTS('',3,(#7549,#7550,#7551,#7552,#7553,#7554,
#7555,#7556,#7557,#7558,#7559,#7560),.UNSPECIFIED.,.F.,.F.,(4,2,2,2,2,4),
(-0.362871505646336,-0.274155479863949,-0.18271451894341,-0.100676077089741,
-0.0480731533577358,-4.69376613687622E-8),.UNSPECIFIED.);
#1386=B_SPLINE_CURVE_WITH_KNOTS('',3,(#7563,#7564,#7565,#7566,#7567,#7568,
#7569,#7570,#7571,#7572,#7573,#7574),.UNSPECIFIED.,.F.,.F.,(4,2,2,2,2,4),
(-0.365098439792926,-0.316918710131062,-0.264213937899729,-0.181785743458761,
-0.0898914967914955,-9.99999990813905E-7),.UNSPECIFIED.);
#1387=B_SPLINE_CURVE_WITH_KNOTS('',3,(#7584,#7585,#7586,#7587,#7588,#7589,
#7590,#7591,#7592,#7593,#7594,#7595),.UNSPECIFIED.,.F.,.F.,(4,2,2,2,2,4),
(-0.362884032462414,-0.274132691310732,-0.182717829525349,-0.100688494943236,
-0.0480786317165661,0.),.UNSPECIFIED.);
#1388=B_SPLINE_CURVE_WITH_KNOTS('',3,(#7598,#7599,#7600,#7601,#7602,#7603,
#7604,#7605,#7606,#7607,#7608,#7609),.UNSPECIFIED.,.F.,.F.,(4,2,2,2,2,4),
(-0.365096305665182,-0.31691825532505,-0.264216003972505,-0.181784730484854,
-0.0898741884806459,-9.99999991813105E-7),.UNSPECIFIED.);
#1389=B_SPLINE_CURVE_WITH_KNOTS('',3,(#7612,#7613,#7614,#7615,#7616,#7617,
#7618,#7619,#7620,#7621,#7622,#7623,#7624,#7625,#7626,#7627,#7628,#7629,
#7630,#7631,#7632,#7633,#7634,#7635,#7636,#7637,#7638,#7639,#7640,#7641,
#7642,#7643,#7644,#7645,#7646,#7647,#7648,#7649,#7650,#7651,#7652,#7653,
#7654,#7655,#7656,#7657,#7658,#7659,#7660,#7661,#7662,#7663,#7664,#7665,
#7666,#7667,#7668,#7669,#7670,#7671,#7672,#7673,#7674,#7675,#7676,#7677,
#7678,#7679,#7680,#7681,#7682,#7683,#7684,#7685,#7686,#7687,#7688,#7689,
#7690,#7691,#7692,#7693,#7694,#7695,#7696,#7697,#7698,#7699),
 .UNSPECIFIED.,.F.,.F.,(4,3,3,3,3,3,3,3,3,3,3,3,3,3,3,3,3,3,3,3,3,3,3,3,
3,3,3,3,3,4),(1.38777878078145E-17,0.000399606416623122,0.00129850035904466,
0.00137933684600951,0.00158113969895516,0.00218306995011964,0.00236541975885409,
0.00237170954843273,0.0031622793979103,0.00420324675762938,0.00433750131101735,
0.00474341909686545,0.00532262963062005,0.0060793421404212,0.00630880058678835,
0.00632455879582059,0.00729497563368212,0.00790569849477573,0.00828085431408244,
0.00869626834425331,0.00921480780263691,0.00926713505608969,0.00948683819373088,
0.0102553852467388,0.0109880837570885,0.011067977892686,0.0112448745518984,
0.0117403235766751,0.0122357726014517,0.0126491175916412),.UNSPECIFIED.);
#1390=B_SPLINE_CURVE_WITH_KNOTS('',3,(#7703,#7704,#7705,#7706,#7707,#7708,
#7709,#7710,#7711,#7712),.UNSPECIFIED.,.F.,.F.,(4,2,2,2,4),(-0.917009726243287,
-0.836713680249397,-0.758350426571219,-0.683089589535854,-0.610699399852799),
 .UNSPECIFIED.);
#1391=B_SPLINE_CURVE_WITH_KNOTS('',3,(#7715,#7716,#7717,#7718,#7719,#7720,
#7721,#7722,#7723,#7724),.UNSPECIFIED.,.F.,.F.,(4,2,2,2,4),(-0.610699399852799,
-0.538309210169743,-0.463048373134379,-0.384685119456201,-0.30438907346231),
 .UNSPECIFIED.);
#1392=B_SPLINE_CURVE_WITH_KNOTS('',3,(#7729,#7730,#7731,#7732,#7733,#7734,
#7735,#7736,#7737,#7738,#7739,#7740,#7741,#7742,#7743,#7744,#7745,#7746,
#7747,#7748,#7749,#7750,#7751,#7752,#7753,#7754,#7755,#7756,#7757,#7758,
#7759,#7760,#7761,#7762,#7763,#7764,#7765,#7766,#7767,#7768,#7769,#7770,
#7771,#7772,#7773,#7774,#7775,#7776,#7777,#7778,#7779,#7780,#7781,#7782,
#7783,#7784,#7785,#7786,#7787,#7788,#7789,#7790,#7791,#7792,#7793,#7794,
#7795,#7796,#7797,#7798,#7799,#7800,#7801,#7802,#7803,#7804,#7805,#7806,
#7807,#7808,#7809,#7810),.UNSPECIFIED.,.F.,.F.,(4,3,3,3,3,3,3,3,3,3,3,3,
3,3,3,3,3,3,3,3,3,3,3,3,3,3,3,4),(2.60208521396521E-18,0.000408621230909919,
0.00138092877422375,0.00156984971266035,0.00235477456899053,0.00235698685553903,
0.0031396994253207,0.00333641997351489,0.00420225476883832,0.00431638805279074,
0.00470954913798105,0.00529643442975242,0.00627638074485589,0.0062793988506414,
0.00706432370697158,0.00725654782189099,0.00784924856330175,0.00823639758948238,
0.00863417341963193,0.0092162185048964,0.0094190982759621,0.01003718926061,
0.0101955027955133,0.0102040231322923,0.0109889479886225,0.0111714628099954,
0.0121441014440987,0.0125587977012828),.UNSPECIFIED.);
#1393=B_SPLINE_CURVE_WITH_KNOTS('',3,(#7812,#7813,#7814,#7815,#7816,#7817,
#7818,#7819,#7820,#7821),.UNSPECIFIED.,.F.,.F.,(4,2,2,2,4),(0.30438907346231,
0.384685119456201,0.463048373134379,0.538309210169743,0.610699399852799),
 .UNSPECIFIED.);
#1394=B_SPLINE_CURVE_WITH_KNOTS('',3,(#7824,#7825,#7826,#7827,#7828,#7829,
#7830,#7831,#7832,#7833),.UNSPECIFIED.,.F.,.F.,(4,2,2,2,4),(0.610699399852799,
0.683089589535854,0.758350426571219,0.836713680249397,0.917009726243287),
 .UNSPECIFIED.);
#1395=B_SPLINE_CURVE_WITH_KNOTS('',3,(#7835,#7836,#7837,#7838,#7839,#7840,
#7841,#7842,#7843,#7844,#7845,#7846,#7847,#7848,#7849,#7850,#7851,#7852,
#7853,#7854,#7855,#7856,#7857,#7858,#7859,#7860,#7861,#7862,#7863,#7864,
#7865,#7866,#7867,#7868,#7869,#7870,#7871,#7872,#7873,#7874,#7875,#7876,
#7877,#7878,#7879,#7880,#7881,#7882,#7883,#7884,#7885,#7886,#7887,#7888,
#7889,#7890,#7891,#7892,#7893,#7894,#7895,#7896,#7897,#7898,#7899,#7900,
#7901,#7902,#7903,#7904,#7905,#7906,#7907,#7908,#7909,#7910,#7911,#7912,
#7913,#7914,#7915,#7916,#7917,#7918,#7919),.UNSPECIFIED.,.F.,.F.,(4,3,3,
3,3,3,3,3,3,3,3,3,3,3,3,3,3,3,3,3,3,3,3,3,3,3,3,3,4),(1.30496590065728E-17,
0.000400535898609883,0.000997223897656586,0.00138427158256107,0.00158086386747061,
0.00237117917706769,0.00316172773494121,0.00390531090957887,0.00434542243932705,
0.00474259160241181,0.00524658086419516,0.00533175204143861,0.00553302353614712,
0.00610814380124694,0.00631869508804951,0.00632345546988242,0.00711388740361772,
0.00730535224261997,0.00790431933735302,0.00829245922415217,0.00869475127108832,
0.00927921238445572,0.00948518320482362,0.0102661645794107,0.0110660470722942,
0.0112527819469325,0.0117750630618308,0.0122387403294437,0.0126469109397648),
 .UNSPECIFIED.);
#1396=B_SPLINE_CURVE_WITH_KNOTS('',3,(#7921,#7922,#7923,#7924,#7925,#7926,
#7927,#7928,#7929,#7930),.UNSPECIFIED.,.F.,.F.,(4,2,2,2,4),(-0.917010857974424,
-0.836714811980533,-0.758351558302355,-0.683090721266991,-0.610700531583935),
 .UNSPECIFIED.);
#1397=B_SPLINE_CURVE_WITH_KNOTS('',3,(#7933,#7934,#7935,#7936,#7937,#7938,
#7939,#7940,#7941,#7942),.UNSPECIFIED.,.F.,.F.,(4,2,2,2,4),(-0.610699399852799,
-0.538309210169743,-0.463048373134379,-0.384685119456201,-0.30438907346231),
 .UNSPECIFIED.);
#1398=B_SPLINE_CURVE_WITH_KNOTS('',3,(#7944,#7945,#7946,#7947,#7948,#7949,
#7950,#7951,#7952,#7953,#7954,#7955,#7956,#7957,#7958,#7959,#7960,#7961,
#7962,#7963,#7964,#7965,#7966,#7967,#7968,#7969,#7970,#7971,#7972,#7973,
#7974,#7975,#7976,#7977,#7978,#7979,#7980,#7981,#7982,#7983,#7984,#7985,
#7986,#7987,#7988,#7989,#7990,#7991,#7992,#7993,#7994,#7995,#7996,#7997,
#7998,#7999,#8000,#8001,#8002,#8003,#8004,#8005,#8006,#8007,#8008,#8009,
#8010,#8011,#8012,#8013,#8014,#8015,#8016,#8017,#8018,#8019,#8020,#8021,
#8022,#8023,#8024,#8025,#8026,#8027,#8028,#8029,#8030,#8031),
 .UNSPECIFIED.,.F.,.F.,(4,3,3,3,3,3,3,3,3,3,3,3,3,3,3,3,3,3,3,3,3,3,3,3,
3,3,3,3,3,4),(3.46944695195361E-18,0.000410051165251199,0.00133968420328458,
0.00156655532439467,0.00221186581193398,0.00235693864354504,0.00300597240703075,
0.00313311064878935,0.00360729264710897,0.00391638831098668,0.00431136042835414,
0.00469966597318402,0.00540563368882195,0.00610076794994382,0.00626622129757869,
0.00626747608388259,0.00681315808315167,0.00704949895977602,0.00724549920617735,
0.00775072389761868,0.00783277662197336,0.00822300176904177,0.00920143005432391,
0.00939933194636803,0.010179032653128,0.0101826096085654,0.0109658872707627,
0.0111531106855899,0.0121225856750134,0.0125324425951574),.UNSPECIFIED.);
#1399=B_SPLINE_CURVE_WITH_KNOTS('',3,(#8033,#8034,#8035,#8036,#8037,#8038,
#8039,#8040,#8041,#8042),.UNSPECIFIED.,.F.,.F.,(4,2,2,2,4),(0.30438907346231,
0.384685119456201,0.463048373134379,0.538309210169743,0.610699399852799),
 .UNSPECIFIED.);
#1400=B_SPLINE_CURVE_WITH_KNOTS('',3,(#8045,#8046,#8047,#8048,#8049,#8050,
#8051,#8052,#8053,#8054),.UNSPECIFIED.,.F.,.F.,(4,2,2,2,4),(0.610699399852799,
0.683089589535855,0.758350426571219,0.836713680249397,0.917009726243288),
 .UNSPECIFIED.);
#1401=B_SPLINE_CURVE_WITH_KNOTS('',3,(#8057,#8058,#8059,#8060,#8061,#8062,
#8063,#8064,#8065,#8066,#8067,#8068,#8069,#8070,#8071,#8072,#8073,#8074,
#8075,#8076,#8077,#8078,#8079,#8080,#8081,#8082,#8083,#8084,#8085,#8086,
#8087,#8088,#8089,#8090,#8091,#8092,#8093,#8094,#8095,#8096,#8097,#8098,
#8099,#8100,#8101,#8102,#8103,#8104,#8105,#8106,#8107,#8108,#8109,#8110,
#8111,#8112,#8113,#8114,#8115,#8116,#8117,#8118,#8119,#8120,#8121,#8122,
#8123,#8124,#8125,#8126,#8127,#8128,#8129,#8130,#8131,#8132,#8133,#8134,
#8135,#8136,#8137,#8138,#8139,#8140,#8141,#8142,#8143,#8144,#8145,#8146,
#8147),.UNSPECIFIED.,.F.,.F.,(4,3,3,3,3,3,3,3,3,3,3,3,3,3,3,3,3,3,3,3,3,
3,3,3,3,3,3,3,3,3,4),(1.73472347597681E-18,0.00039988746592532,0.00129491695484595,
0.00137824963045728,0.00157959224294063,0.00221817566303284,0.00236299587550376,
0.00236938836441095,0.00315918448588126,0.00334829919727405,0.00433350078435649,
0.00473877672882189,0.00531878197917401,0.00552857285029221,0.00621168871910692,
0.00630402471854614,0.00631836897176252,0.00700327686816661,0.00728961045190966,
0.00789796121470315,0.00827440785064211,0.00868775733617347,0.0091828676285263,
0.00926005766828055,0.00947755345764378,0.0102465428671901,0.0110571457005844,
0.0112335337469168,0.0117819684897293,0.0122215199127025,0.012636737943525),
 .UNSPECIFIED.);
#1402=B_SPLINE_CURVE_WITH_KNOTS('',3,(#8151,#8152,#8153,#8154,#8155,#8156,
#8157,#8158,#8159,#8160),.UNSPECIFIED.,.F.,.F.,(4,2,2,2,4),(-0.917009726243287,
-0.836713680249397,-0.758350426571219,-0.683089589535854,-0.610699399852799),
 .UNSPECIFIED.);
#1403=B_SPLINE_CURVE_WITH_KNOTS('',3,(#8163,#8164,#8165,#8166,#8167,#8168,
#8169,#8170,#8171,#8172),.UNSPECIFIED.,.F.,.F.,(4,2,2,2,4),(-0.610699399852799,
-0.538309210169743,-0.463048373134379,-0.384685119456201,-0.30438907346231),
 .UNSPECIFIED.);
#1404=B_SPLINE_CURVE_WITH_KNOTS('',3,(#8177,#8178,#8179,#8180,#8181,#8182,
#8183,#8184,#8185,#8186,#8187,#8188,#8189,#8190,#8191,#8192,#8193,#8194,
#8195,#8196,#8197,#8198,#8199,#8200,#8201,#8202,#8203,#8204,#8205,#8206,
#8207,#8208,#8209,#8210,#8211,#8212,#8213,#8214,#8215,#8216,#8217,#8218,
#8219,#8220,#8221,#8222,#8223,#8224,#8225,#8226,#8227,#8228,#8229,#8230,
#8231,#8232,#8233,#8234,#8235,#8236,#8237,#8238,#8239,#8240,#8241,#8242,
#8243,#8244,#8245,#8246,#8247,#8248,#8249,#8250,#8251,#8252,#8253,#8254,
#8255,#8256,#8257,#8258,#8259,#8260,#8261),.UNSPECIFIED.,.F.,.F.,(4,3,3,
3,3,3,3,3,3,3,3,3,3,3,3,3,3,3,3,3,3,3,3,3,3,3,3,3,4),(6.07153216591882E-18,
0.00040720230965342,0.00137997790341395,0.00157140084496842,0.0023570743820119,
0.00235710126745262,0.00314280168993683,0.00333751194950876,0.00416238965998517,
0.00431851263176076,0.00471420253490524,0.00529977060133669,0.0062805746484409,
0.00628560337987365,0.00707130380235786,0.00726149881588422,0.00785700422484207,
0.00824263329795796,0.00864270464732627,0.00917430501847767,0.00922314347734942,
0.00942840506981048,0.00998906064805868,0.0102032494512671,0.0102141054922947,
0.0109998059147789,0.0119266401717515,0.0121550490383017,0.0125712067597473),
 .UNSPECIFIED.);
#1405=B_SPLINE_CURVE_WITH_KNOTS('',3,(#8263,#8264,#8265,#8266,#8267,#8268,
#8269,#8270,#8271,#8272),.UNSPECIFIED.,.F.,.F.,(4,2,2,2,4),(0.30438907346231,
0.384685119456201,0.463048373134379,0.538309210169743,0.610699399852799),
 .UNSPECIFIED.);
#1406=B_SPLINE_CURVE_WITH_KNOTS('',3,(#8275,#8276,#8277,#8278,#8279,#8280,
#8281,#8282,#8283,#8284),.UNSPECIFIED.,.F.,.F.,(4,2,2,2,4),(0.610699399852799,
0.683089589535855,0.758350426571219,0.836713680249397,0.917009726243288),
 .UNSPECIFIED.);
#1407=B_SPLINE_CURVE_WITH_KNOTS('',3,(#8288,#8289,#8290,#8291,#8292,#8293,
#8294,#8295,#8296,#8297),.UNSPECIFIED.,.F.,.F.,(4,1,1,1,1,1,1,4),(1.30100171735751E-9,
0.0016146554249922,0.00242198313748831,0.00322931084998441,0.00403663856248051,
0.00484396627497661,0.00565129398747271,0.00645802980103412),
 .UNSPECIFIED.);
#1408=B_SPLINE_CURVE_WITH_KNOTS('',3,(#8301,#8302,#8303,#8304,#8305,#8306,
#8307,#8308,#8309,#8310,#8311,#8312,#8313,#8314,#8315,#8316,#8317,#8318,
#8319,#8320,#8321,#8322,#8323,#8324,#8325,#8326,#8327,#8328,#8329,#8330,
#8331,#8332,#8333,#8334,#8335,#8336,#8337,#8338,#8339,#8340,#8341,#8342,
#8343,#8344,#8345,#8346,#8347,#8348,#8349,#8350,#8351,#8352),
 .UNSPECIFIED.,.F.,.F.,(4,3,3,3,3,3,3,3,3,3,3,3,3,3,3,3,3,4),(0.00648543634797121,
0.0064967267157505,0.00649946849415933,0.00731190205592925,0.00731946089640744,
0.00812433561769917,0.00814225039785811,0.00893676917946909,0.00896508534539126,
0.009749202741239,0.00978815035523349,0.010612333053574,0.0113740698647788,
0.0114378447184054,0.0119000363007037,0.0122657233205253,0.0127116726794121,
0.0129989369883187),.UNSPECIFIED.);
#1409=B_SPLINE_CURVE_WITH_KNOTS('',3,(#8356,#8357,#8358,#8359,#8360,#8361,
#8362,#8363,#8364,#8365,#8366),.UNSPECIFIED.,.F.,.F.,(4,1,1,1,1,1,1,1,4),
(6.42162746646723E-10,0.000808623423577319,0.00161724684715464,0.00242587027073195,
0.00323449369430927,0.00404311711788659,0.00485174054146391,0.00566036396504123,
0.00646652117894175),.UNSPECIFIED.);
#1410=B_SPLINE_CURVE_WITH_KNOTS('',3,(#8369,#8370,#8371,#8372,#8373,#8374,
#8375,#8376,#8377,#8378,#8379,#8380,#8381,#8382,#8383,#8384,#8385,#8386,
#8387,#8388,#8389,#8390,#8391,#8392,#8393,#8394,#8395,#8396,#8397,#8398,
#8399,#8400,#8401,#8402,#8403,#8404,#8405,#8406,#8407,#8408,#8409,#8410,
#8411,#8412,#8413,#8414,#8415,#8416,#8417,#8418,#8419,#8420,#8421,#8422,
#8423),.UNSPECIFIED.,.F.,.F.,(4,3,3,3,3,3,3,3,3,3,3,3,3,3,3,3,3,3,4),(0.00647004505939142,
0.00647363968946843,0.00647720040263265,0.00728284465065198,0.00729848964174994,
0.00801241832704487,0.00809204961183553,0.00811990123016667,0.00894157646616379,
0.00971045953420264,0.00976287368659868,0.010321243105252,0.0105196644953862,
0.0105845039445962,0.011274043522722,0.0113288694565697,0.0114042476736799,
0.0124870589427851,0.0129472785059492),.UNSPECIFIED.);
#1411=B_SPLINE_CURVE_WITH_KNOTS('',3,(#8425,#8426,#8427,#8428,#8429,#8430,
#8431,#8432,#8433,#8434),.UNSPECIFIED.,.F.,.F.,(4,1,1,1,1,1,1,4),(0.,0.000811969399540441,
0.00162393879908088,0.00324787759816176,0.0040598469977022,0.00487181639724265,
0.00568378579678309,0.00648320241242164),.UNSPECIFIED.);
#1412=B_SPLINE_CURVE_WITH_KNOTS('',3,(#8437,#8438,#8439,#8440,#8441,#8442,
#8443,#8444,#8445,#8446,#8447,#8448,#8449,#8450,#8451,#8452,#8453,#8454,
#8455,#8456,#8457,#8458,#8459,#8460,#8461,#8462,#8463,#8464,#8465,#8466,
#8467,#8468,#8469,#8470,#8471,#8472,#8473,#8474,#8475,#8476,#8477,#8478,
#8479,#8480,#8481,#8482,#8483,#8484,#8485,#8486,#8487,#8488,#8489,#8490,
#8491,#8492,#8493,#8494),.UNSPECIFIED.,.F.,.F.,(4,3,3,3,3,3,3,3,3,3,3,3,
3,3,3,3,3,3,3,4),(0.00648198680776405,0.0064936104430031,0.00649369947494339,
0.00730541190931131,0.00731614940961611,0.00811712434367923,0.00813876531642026,
0.00892883677804716,0.00896138011049144,0.00974054921241508,0.00978423042042142,
0.010486564667016,0.010552261646783,0.0106072334779918,0.0113639740811509,
0.0114307075734888,0.011991699677843,0.012255239290347,0.012808829510336,
0.0129873989498868),.UNSPECIFIED.);
#1413=B_SPLINE_CURVE_WITH_KNOTS('',3,(#8496,#8497,#8498,#8499,#8500,#8501,
#8502,#8503,#8504,#8505,#8506,#8507,#8508,#8509,#8510,#8511,#8512,#8513,
#8514,#8515,#8516,#8517,#8518,#8519,#8520,#8521,#8522,#8523,#8524,#8525,
#8526,#8527,#8528,#8529,#8530,#8531,#8532,#8533,#8534,#8535,#8536,#8537,
#8538),.UNSPECIFIED.,.F.,.F.,(4,3,3,3,3,3,3,3,3,3,3,3,3,3,4),(9.63404319765764E-10,
0.000487198195571319,0.000809509611833977,0.00122696048983144,0.00161901922366795,
0.00219920987370979,0.00278322336955574,0.00323803844733591,0.00371315641008233,
0.00404754805916988,0.00445496587286083,0.00485705767100386,0.0055156033353318,
0.00617364200047874,0.0064717827093511),.UNSPECIFIED.);
#1414=B_SPLINE_CURVE_WITH_KNOTS('',3,(#8541,#8542,#8543,#8544,#8545,#8546,
#8547,#8548,#8549,#8550,#8551,#8552,#8553,#8554,#8555,#8556,#8557,#8558,
#8559,#8560,#8561,#8562,#8563,#8564,#8565,#8566,#8567,#8568,#8569,#8570,
#8571,#8572,#8573,#8574,#8575,#8576,#8577,#8578,#8579,#8580,#8581,#8582,
#8583,#8584,#8585,#8586,#8587,#8588,#8589),.UNSPECIFIED.,.F.,.F.,(4,3,3,
3,3,3,3,3,3,3,3,3,3,3,3,3,4),(0.0064898095819301,0.00649606092685136,0.00698916367409277,
0.00748291484157417,0.00797566710589656,0.0081200761585642,0.00857341799443063,
0.00902647257612117,0.00947992094581784,0.00974409139027704,0.0102520995680632,
0.0107611012391323,0.0112695579712555,0.0113681066219899,0.0119417158433385,
0.012514860767218,0.0129921218537027),.UNSPECIFIED.);
#1415=B_SPLINE_CURVE_WITH_KNOTS('',3,(#8590,#8591,#8592,#8593,#8594,#8595,
#8596,#8597,#8598,#8599,#8600,#8601,#8602,#8603,#8604,#8605,#8606,#8607,
#8608,#8609,#8610,#8611,#8612,#8613,#8614,#8615,#8616,#8617,#8618,#8619,
#8620,#8621,#8622,#8623,#8624,#8625,#8626,#8627,#8628,#8629,#8630,#8631,
#8632,#8633,#8634,#8635),.UNSPECIFIED.,.F.,.F.,(4,3,3,3,3,3,3,3,3,3,3,3,
3,3,3,4),(0.,0.000604609839358999,0.00121565628960328,0.00162401523171284,
0.00216471951290587,0.00243602284756926,0.00310314498849404,0.00324803046342568,
0.00365403427135389,0.0040600380792821,0.00451926183054206,0.00487204569513852,
0.00535427083414837,0.00583643300319355,0.0063191303600972,0.0064898095819301),
 .UNSPECIFIED.);
#1416=B_SPLINE_CURVE_WITH_KNOTS('',3,(#8636,#8637,#8638,#8639,#8640,#8641,
#8642,#8643,#8644,#8645,#8646,#8647,#8648,#8649,#8650,#8651,#8652,#8653,
#8654,#8655,#8656,#8657,#8658,#8659,#8660,#8661,#8662,#8663,#8664,#8665,
#8666,#8667,#8668,#8669,#8670,#8671,#8672,#8673,#8674,#8675,#8676,#8677,
#8678,#8679,#8680,#8681),.UNSPECIFIED.,.F.,.F.,(4,3,3,3,3,3,3,3,3,3,3,3,
3,3,3,4),(0.0064717827093511,0.00647607689467181,0.0068808317005888,0.00728558650650579,
0.00779796951019886,0.00809509611833977,0.00863663393440084,0.00917632462956808,
0.00971411534200772,0.0101188701479247,0.0105236249538417,0.0110729177361821,
0.0113331345656757,0.0119056167126292,0.0124755694459539,0.0129521530063804),
 .UNSPECIFIED.);
#1417=B_SPLINE_CURVE_WITH_KNOTS('',3,(#8682,#8683,#8684,#8685,#8686,#8687,
#8688,#8689,#8690,#8691,#8692,#8693,#8694,#8695,#8696,#8697,#8698,#8699,
#8700,#8701,#8702,#8703,#8704,#8705,#8706,#8707,#8708,#8709,#8710,#8711,
#8712,#8713,#8714,#8715,#8716,#8717,#8718,#8719,#8720,#8721,#8722,#8723,
#8724,#8725,#8726,#8727,#8728,#8729,#8730,#8731,#8732,#8733),
 .UNSPECIFIED.,.F.,.F.,(4,3,3,3,3,3,3,3,3,3,3,3,3,3,3,3,3,4),(0.,0.000490776775537461,
0.00073393694656371,0.00124207968922223,0.00155724861738079,0.00162342486873585,
0.00247225450565376,0.00320323287865645,0.00324684973747169,0.00392447218817879,
0.00402584241665628,0.00405856217183962,0.00480782344391585,0.00484857865525814,
0.00487027460620754,0.00567112301456725,0.00568198704057546,0.00648198680776405),
 .UNSPECIFIED.);
#1418=B_SPLINE_CURVE_WITH_KNOTS('',3,(#8735,#8736,#8737,#8738,#8739,#8740,
#8741,#8742,#8743,#8744,#8745),.UNSPECIFIED.,.F.,.F.,(4,1,1,1,1,1,1,1,4),
(0.00648320241242164,0.00649575519632353,0.00730772459586397,0.00811969399540441,
0.00893166339494485,0.00974363279448529,0.0105556021940257,0.0113675715935662,
0.0129915103926471),.UNSPECIFIED.);
#1419=B_SPLINE_CURVE_WITH_KNOTS('',3,(#8748,#8749,#8750,#8751,#8752,#8753,
#8754,#8755,#8756,#8757,#8758,#8759,#8760,#8761,#8762,#8763,#8764,#8765,
#8766,#8767,#8768,#8769,#8770,#8771,#8772,#8773,#8774,#8775,#8776,#8777,
#8778,#8779,#8780,#8781,#8782,#8783,#8784,#8785,#8786,#8787,#8788,#8789,
#8790,#8791,#8792,#8793,#8794,#8795,#8796,#8797,#8798,#8799,#8800,#8801,
#8802),.UNSPECIFIED.,.F.,.F.,(4,3,3,3,3,3,3,3,3,3,3,3,3,3,3,3,3,3,4),(9.20377798281372E-10,
0.000670048056992883,0.000728118409870351,0.000809204961183555,0.00135514668727475,
0.00154786083600147,0.00161840992236711,0.00219729439487813,0.00236979743471876,
0.00242761488355066,0.0031915074931542,0.00323681984473421,0.00401314180766438,
0.00404602480591777,0.00483449084074671,0.00485522976710132,0.00565589261146122,
0.00566443472828487,0.00647004505939142),.UNSPECIFIED.);
#1420=B_SPLINE_CURVE_WITH_KNOTS('',3,(#8803,#8804,#8805,#8806,#8807,#8808,
#8809,#8810,#8811,#8812),.UNSPECIFIED.,.F.,.F.,(4,1,1,1,1,1,1,4),(0.00646652117894175,
0.00646898738861854,0.00727761081219586,0.00808623423577318,0.00970348108292781,
0.0105121045065051,0.0113207279300824,0.0129379736427185),.UNSPECIFIED.);
#1421=B_SPLINE_CURVE_WITH_KNOTS('',3,(#8813,#8814,#8815,#8816,#8817,#8818,
#8819,#8820,#8821,#8822,#8823,#8824,#8825,#8826,#8827,#8828,#8829,#8830,
#8831,#8832,#8833,#8834,#8835,#8836,#8837,#8838,#8839,#8840,#8841,#8842,
#8843,#8844,#8845,#8846,#8847,#8848,#8849,#8850,#8851,#8852,#8853,#8854,
#8855,#8856,#8857,#8858),.UNSPECIFIED.,.F.,.F.,(4,3,3,3,3,3,3,3,3,3,3,3,
3,3,3,4),(0.,0.0004185116728278,0.000735801334826299,0.000812433561769917,
0.00155917246295599,0.00162486712353983,0.00238263123545803,0.00320564025005124,
0.00324973424707967,0.00402847232243131,0.00406216780884958,0.00485131517672913,
0.0048746013706195,0.00567403038972561,0.00568703493238942,0.00648543634797121),
 .UNSPECIFIED.);
#1422=B_SPLINE_CURVE_WITH_KNOTS('',3,(#8859,#8860,#8861,#8862,#8863,#8864,
#8865,#8866,#8867,#8868),.UNSPECIFIED.,.F.,.F.,(4,1,1,1,1,1,1,4),(0.00645802980103412,
0.00645862169996881,0.00726594941246491,0.00807327712496101,0.00968793254995321,
0.0104952602624493,0.0113025879749454,0.0129172416014509),.UNSPECIFIED.);
#1423=B_SPLINE_CURVE_WITH_KNOTS('',3,(#8871,#8872,#8873,#8874,#8875,#8876,
#8877,#8878,#8879,#8880,#8881,#8882),.UNSPECIFIED.,.F.,.F.,(4,2,2,2,2,4),
(-0.362871564393025,-0.274154813883086,-0.182714570720302,-0.100676259181141,
-0.0480732761959632,-4.4821511446802E-8),.UNSPECIFIED.);
#1424=B_SPLINE_CURVE_WITH_KNOTS('',3,(#8883,#8884,#8885,#8886,#8887,#8888,
#8889,#8890,#8891,#8892,#8893,#8894),.UNSPECIFIED.,.F.,.F.,(4,2,2,2,2,4),
(-0.365095457281969,-0.316915096094452,-0.264209783934842,-0.181784066815884,
-0.0898944546920999,-9.99999993344656E-7),.UNSPECIFIED.);
#1425=B_SPLINE_CURVE_WITH_KNOTS('',3,(#8897,#8898,#8899,#8900,#8901,#8902,
#8903,#8904,#8905,#8906,#8907,#8908),.UNSPECIFIED.,.F.,.F.,(4,2,2,2,2,4),
(-0.362873161532576,-0.274151352800392,-0.182714900485669,-0.100677632331331,
-0.0480739883883429,-3.14822323210784E-8),.UNSPECIFIED.);
#1426=B_SPLINE_CURVE_WITH_KNOTS('',3,(#8909,#8910,#8911,#8912,#8913,#8914,
#8915,#8916,#8917,#8918,#8919,#8920),.UNSPECIFIED.,.F.,.F.,(4,2,2,2,2,4),
(-0.365090467953361,-0.316909793473234,-0.264204439712853,-0.18178222731987,
-0.0898981188055125,-9.99999993270273E-7),.UNSPECIFIED.);
#1584=CIRCLE('',#4330,18.);
#1585=CIRCLE('',#4331,71.);
#1586=CIRCLE('',#4333,18.);
#1587=CIRCLE('',#4334,71.);
#1588=CIRCLE('',#4335,71.);
#1589=CIRCLE('',#4337,18.);
#1590=CIRCLE('',#4338,71.);
#1591=CIRCLE('',#4340,18.);
#1592=CIRCLE('',#4341,71.);
#1593=CIRCLE('',#4342,71.);
#1594=CIRCLE('',#4344,18.);
#1595=CIRCLE('',#4345,71.);
#1596=CIRCLE('',#4347,18.);
#1597=CIRCLE('',#4348,71.);
#1598=CIRCLE('',#4356,10.);
#1599=CIRCLE('',#4357,69.);
#1600=CIRCLE('',#4358,71.);
#1601=CIRCLE('',#4359,69.);
#1602=CIRCLE('',#4360,69.);
#1603=CIRCLE('',#4361,69.);
#1604=CIRCLE('',#4362,71.);
#1605=CIRCLE('',#4364,18.);
#1606=CIRCLE('',#4366,18.);
#1607=CIRCLE('',#4368,16.);
#1608=CIRCLE('',#4369,16.);
#1609=CIRCLE('',#4370,16.);
#1610=CIRCLE('',#4371,16.);
#1611=CIRCLE('',#4372,16.);
#1612=CIRCLE('',#4373,16.);
#1613=CIRCLE('',#4374,16.);
#1614=CIRCLE('',#4375,16.);
#1615=CIRCLE('',#4376,16.);
#1616=CIRCLE('',#4377,16.);
#1617=CIRCLE('',#4378,16.);
#1618=CIRCLE('',#4379,16.);
#1862=VERTEX_POINT('',#7170);
#1863=VERTEX_POINT('',#7171);
#1864=VERTEX_POINT('',#7173);
#1865=VERTEX_POINT('',#7262);
#1866=VERTEX_POINT('',#7264);
#1867=VERTEX_POINT('',#7275);
#1868=VERTEX_POINT('',#7288);
#1869=VERTEX_POINT('',#7289);
#1870=VERTEX_POINT('',#7291);
#1871=VERTEX_POINT('',#7383);
#1872=VERTEX_POINT('',#7385);
#1873=VERTEX_POINT('',#7396);
#1874=VERTEX_POINT('',#7410);
#1875=VERTEX_POINT('',#7423);
#1876=VERTEX_POINT('',#7438);
#1877=VERTEX_POINT('',#7439);
#1878=VERTEX_POINT('',#7441);
#1879=VERTEX_POINT('',#7443);
#1880=VERTEX_POINT('',#7445);
#1881=VERTEX_POINT('',#7458);
#1882=VERTEX_POINT('',#7460);
#1883=VERTEX_POINT('',#7475);
#1884=VERTEX_POINT('',#7476);
#1885=VERTEX_POINT('',#7478);
#1886=VERTEX_POINT('',#7480);
#1887=VERTEX_POINT('',#7482);
#1888=VERTEX_POINT('',#7495);
#1889=VERTEX_POINT('',#7510);
#1890=VERTEX_POINT('',#7511);
#1891=VERTEX_POINT('',#7513);
#1892=VERTEX_POINT('',#7515);
#1893=VERTEX_POINT('',#7517);
#1894=VERTEX_POINT('',#7530);
#1895=VERTEX_POINT('',#7532);
#1896=VERTEX_POINT('',#7548);
#1897=VERTEX_POINT('',#7561);
#1898=VERTEX_POINT('',#7576);
#1899=VERTEX_POINT('',#7577);
#1900=VERTEX_POINT('',#7579);
#1901=VERTEX_POINT('',#7581);
#1902=VERTEX_POINT('',#7583);
#1903=VERTEX_POINT('',#7596);
#1904=VERTEX_POINT('',#7611);
#1905=VERTEX_POINT('',#7700);
#1906=VERTEX_POINT('',#7702);
#1907=VERTEX_POINT('',#7713);
#1908=VERTEX_POINT('',#7726);
#1909=VERTEX_POINT('',#7727);
#1910=VERTEX_POINT('',#7811);
#1911=VERTEX_POINT('',#7822);
#1912=VERTEX_POINT('',#7920);
#1913=VERTEX_POINT('',#7931);
#1914=VERTEX_POINT('',#8032);
#1915=VERTEX_POINT('',#8043);
#1916=VERTEX_POINT('',#8056);
#1917=VERTEX_POINT('',#8148);
#1918=VERTEX_POINT('',#8150);
#1919=VERTEX_POINT('',#8161);
#1920=VERTEX_POINT('',#8174);
#1921=VERTEX_POINT('',#8175);
#1922=VERTEX_POINT('',#8262);
#1923=VERTEX_POINT('',#8273);
#1924=VERTEX_POINT('',#8287);
#1925=VERTEX_POINT('',#8298);
#1926=VERTEX_POINT('',#8300);
#1927=VERTEX_POINT('',#8353);
#1928=VERTEX_POINT('',#8355);
#1929=VERTEX_POINT('',#8367);
#1930=VERTEX_POINT('',#8424);
#1931=VERTEX_POINT('',#8435);
#1932=VERTEX_POINT('',#8495);
#1933=VERTEX_POINT('',#8539);
#1934=VERTEX_POINT('',#8734);
#1935=VERTEX_POINT('',#8746);
#1936=VERTEX_POINT('',#8922);
#1937=VERTEX_POINT('',#8924);
#1938=VERTEX_POINT('',#8927);
#1939=VERTEX_POINT('',#8929);
#1940=VERTEX_POINT('',#8941);
#1941=VERTEX_POINT('',#8942);
#1942=VERTEX_POINT('',#8944);
#1943=VERTEX_POINT('',#8946);
#1944=VERTEX_POINT('',#8950);
#1945=VERTEX_POINT('',#8951);
#1946=VERTEX_POINT('',#8953);
#1947=VERTEX_POINT('',#8955);
#2334=EDGE_CURVE('',#1862,#1863,#504,.T.);
#2335=EDGE_CURVE('',#1863,#1864,#1371,.T.);
#2336=EDGE_CURVE('',#1864,#1865,#505,.T.);
#2337=EDGE_CURVE('',#1865,#1866,#1372,.T.);
#2338=EDGE_CURVE('',#1866,#1867,#506,.T.);
#2339=EDGE_CURVE('',#1867,#1862,#1373,.T.);
#2340=EDGE_CURVE('',#1868,#1869,#507,.T.);
#2341=EDGE_CURVE('',#1868,#1870,#1374,.T.);
#2342=EDGE_CURVE('',#1871,#1870,#508,.T.);
#2343=EDGE_CURVE('',#1871,#1872,#1375,.T.);
#2344=EDGE_CURVE('',#1873,#1872,#509,.T.);
#2345=EDGE_CURVE('',#1873,#1869,#1376,.T.);
#2346=EDGE_CURVE('',#1869,#1865,#1584,.T.);
#2347=EDGE_CURVE('',#1864,#1874,#1377,.T.);
#2348=EDGE_CURVE('',#1874,#1875,#1585,.T.);
#2349=EDGE_CURVE('',#1875,#1868,#1378,.T.);
#2350=EDGE_CURVE('',#1876,#1877,#510,.T.);
#2351=EDGE_CURVE('',#1876,#1878,#1586,.T.);
#2352=EDGE_CURVE('',#1878,#1879,#511,.T.);
#2353=EDGE_CURVE('',#1879,#1880,#1379,.T.);
#2354=EDGE_CURVE('',#1880,#1881,#1587,.T.);
#2355=EDGE_CURVE('',#1881,#1882,#1588,.T.);
#2356=EDGE_CURVE('',#1882,#1877,#1380,.T.);
#2357=EDGE_CURVE('',#1883,#1884,#512,.T.);
#2358=EDGE_CURVE('',#1883,#1885,#1589,.T.);
#2359=EDGE_CURVE('',#1885,#1886,#513,.T.);
#2360=EDGE_CURVE('',#1886,#1887,#1381,.T.);
#2361=EDGE_CURVE('',#1887,#1888,#1590,.T.);
#2362=EDGE_CURVE('',#1888,#1884,#1382,.T.);
#2363=EDGE_CURVE('',#1889,#1890,#514,.T.);
#2364=EDGE_CURVE('',#1890,#1891,#1591,.T.);
#2365=EDGE_CURVE('',#1892,#1891,#515,.T.);
#2366=EDGE_CURVE('',#1892,#1893,#1383,.T.);
#2367=EDGE_CURVE('',#1893,#1894,#1592,.T.);
#2368=EDGE_CURVE('',#1894,#1895,#1593,.T.);
#2369=EDGE_CURVE('',#1895,#1889,#1384,.T.);
#2370=EDGE_CURVE('',#1862,#1871,#1594,.T.);
#2371=EDGE_CURVE('',#1870,#1896,#1385,.T.);
#2372=EDGE_CURVE('',#1896,#1897,#1595,.T.);
#2373=EDGE_CURVE('',#1897,#1863,#1386,.T.);
#2374=EDGE_CURVE('',#1898,#1899,#516,.T.);
#2375=EDGE_CURVE('',#1898,#1900,#1596,.T.);
#2376=EDGE_CURVE('',#1900,#1901,#517,.T.);
#2377=EDGE_CURVE('',#1901,#1902,#1387,.T.);
#2378=EDGE_CURVE('',#1902,#1903,#1597,.T.);
#2379=EDGE_CURVE('',#1903,#1899,#1388,.T.);
#2380=EDGE_CURVE('',#1884,#1904,#1389,.T.);
#2381=EDGE_CURVE('',#1904,#1905,#518,.T.);
#2382=EDGE_CURVE('',#1905,#1906,#1390,.T.);
#2383=EDGE_CURVE('',#1906,#1907,#519,.F.);
#2384=EDGE_CURVE('',#1907,#1883,#1391,.T.);
#2385=EDGE_CURVE('',#1908,#1909,#520,.T.);
#2386=EDGE_CURVE('',#1908,#1886,#1392,.T.);
#2387=EDGE_CURVE('',#1885,#1910,#1393,.T.);
#2388=EDGE_CURVE('',#1911,#1910,#521,.F.);
#2389=EDGE_CURVE('',#1911,#1909,#1394,.T.);
#2390=EDGE_CURVE('',#1877,#1892,#1395,.T.);
#2391=EDGE_CURVE('',#1891,#1912,#1396,.T.);
#2392=EDGE_CURVE('',#1912,#1913,#522,.F.);
#2393=EDGE_CURVE('',#1913,#1876,#1397,.T.);
#2394=EDGE_CURVE('',#1889,#1879,#1398,.T.);
#2395=EDGE_CURVE('',#1878,#1914,#1399,.T.);
#2396=EDGE_CURVE('',#1915,#1914,#523,.F.);
#2397=EDGE_CURVE('',#1915,#1890,#1400,.T.);
#2398=EDGE_CURVE('',#1899,#1916,#1401,.T.);
#2399=EDGE_CURVE('',#1916,#1917,#524,.T.);
#2400=EDGE_CURVE('',#1917,#1918,#1402,.T.);
#2401=EDGE_CURVE('',#1918,#1919,#525,.T.);
#2402=EDGE_CURVE('',#1919,#1898,#1403,.T.);
#2403=EDGE_CURVE('',#1920,#1921,#526,.T.);
#2404=EDGE_CURVE('',#1920,#1901,#1404,.T.);
#2405=EDGE_CURVE('',#1900,#1922,#1405,.T.);
#2406=EDGE_CURVE('',#1923,#1922,#527,.T.);
#2407=EDGE_CURVE('',#1923,#1921,#1406,.T.);
#2408=EDGE_CURVE('',#1894,#1881,#1598,.T.);
#2409=EDGE_CURVE('',#1893,#1924,#1407,.T.);
#2410=EDGE_CURVE('',#1924,#1925,#1599,.T.);
#2411=EDGE_CURVE('',#1925,#1926,#1408,.T.);
#2412=EDGE_CURVE('',#1927,#1926,#1600,.T.);
#2413=EDGE_CURVE('',#1927,#1928,#1409,.T.);
#2414=EDGE_CURVE('',#1928,#1929,#1601,.T.);
#2415=EDGE_CURVE('',#1929,#1903,#1410,.T.);
#2416=EDGE_CURVE('',#1902,#1930,#1411,.T.);
#2417=EDGE_CURVE('',#1930,#1931,#1602,.T.);
#2418=EDGE_CURVE('',#1931,#1897,#1412,.T.);
#2419=EDGE_CURVE('',#1896,#1932,#1413,.T.);
#2420=EDGE_CURVE('',#1932,#1933,#1603,.T.);
#2421=EDGE_CURVE('',#1933,#1895,#1414,.T.);
#2422=EDGE_CURVE('',#1880,#1933,#1415,.T.);
#2423=EDGE_CURVE('',#1932,#1875,#1416,.T.);
#2424=EDGE_CURVE('',#1874,#1931,#1417,.T.);
#2425=EDGE_CURVE('',#1930,#1934,#1418,.T.);
#2426=EDGE_CURVE('',#1935,#1934,#1604,.T.);
#2427=EDGE_CURVE('',#1935,#1929,#1419,.T.);
#2428=EDGE_CURVE('',#1928,#1888,#1420,.T.);
#2429=EDGE_CURVE('',#1887,#1925,#1421,.T.);
#2430=EDGE_CURVE('',#1924,#1882,#1422,.T.);
#2431=EDGE_CURVE('',#1921,#1917,#1605,.T.);
#2432=EDGE_CURVE('',#1916,#1935,#1423,.T.);
#2433=EDGE_CURVE('',#1934,#1920,#1424,.T.);
#2434=EDGE_CURVE('',#1909,#1905,#1606,.T.);
#2435=EDGE_CURVE('',#1904,#1927,#1425,.T.);
#2436=EDGE_CURVE('',#1926,#1908,#1426,.T.);
#2437=EDGE_CURVE('',#1936,#1936,#1607,.T.);
#2438=EDGE_CURVE('',#1936,#1937,#528,.T.);
#2439=EDGE_CURVE('',#1937,#1915,#1608,.F.);
#2440=EDGE_CURVE('',#1914,#1938,#1609,.F.);
#2441=EDGE_CURVE('',#1938,#1939,#529,.T.);
#2442=EDGE_CURVE('',#1939,#1939,#1610,.T.);
#2443=EDGE_CURVE('',#1938,#1913,#1611,.F.);
#2444=EDGE_CURVE('',#1912,#1937,#1612,.F.);
#2445=EDGE_CURVE('',#1910,#1907,#1613,.F.);
#2446=EDGE_CURVE('',#1906,#1911,#1614,.F.);
#2447=EDGE_CURVE('',#1918,#1923,#1615,.F.);
#2448=EDGE_CURVE('',#1922,#1919,#1616,.F.);
#2449=EDGE_CURVE('',#1872,#1867,#1617,.F.);
#2450=EDGE_CURVE('',#1866,#1873,#1618,.F.);
#2451=EDGE_CURVE('',#1940,#1941,#530,.T.);
#2452=EDGE_CURVE('',#1941,#1942,#531,.T.);
#2453=EDGE_CURVE('',#1942,#1943,#532,.T.);
#2454=EDGE_CURVE('',#1943,#1940,#533,.T.);
#2455=EDGE_CURVE('',#1944,#1945,#534,.T.);
#2456=EDGE_CURVE('',#1946,#1944,#535,.T.);
#2457=EDGE_CURVE('',#1947,#1946,#536,.T.);
#2458=EDGE_CURVE('',#1945,#1947,#537,.T.);
#2459=EDGE_CURVE('',#1941,#1944,#538,.T.);
#2460=EDGE_CURVE('',#1940,#1946,#539,.T.);
#2461=EDGE_CURVE('',#1943,#1947,#540,.T.);
#2462=EDGE_CURVE('',#1942,#1945,#541,.T.);
#3221=ORIENTED_EDGE('',*,*,#2334,.T.);
#3222=ORIENTED_EDGE('',*,*,#2335,.T.);
#3223=ORIENTED_EDGE('',*,*,#2336,.T.);
#3224=ORIENTED_EDGE('',*,*,#2337,.T.);
#3225=ORIENTED_EDGE('',*,*,#2338,.T.);
#3226=ORIENTED_EDGE('',*,*,#2339,.T.);
#3227=ORIENTED_EDGE('',*,*,#2340,.F.);
#3228=ORIENTED_EDGE('',*,*,#2341,.T.);
#3229=ORIENTED_EDGE('',*,*,#2342,.F.);
#3230=ORIENTED_EDGE('',*,*,#2343,.T.);
#3231=ORIENTED_EDGE('',*,*,#2344,.F.);
#3232=ORIENTED_EDGE('',*,*,#2345,.T.);
#3233=ORIENTED_EDGE('',*,*,#2340,.T.);
#3234=ORIENTED_EDGE('',*,*,#2346,.T.);
#3235=ORIENTED_EDGE('',*,*,#2336,.F.);
#3236=ORIENTED_EDGE('',*,*,#2347,.T.);
#3237=ORIENTED_EDGE('',*,*,#2348,.T.);
#3238=ORIENTED_EDGE('',*,*,#2349,.T.);
#3239=ORIENTED_EDGE('',*,*,#2350,.F.);
#3240=ORIENTED_EDGE('',*,*,#2351,.T.);
#3241=ORIENTED_EDGE('',*,*,#2352,.T.);
#3242=ORIENTED_EDGE('',*,*,#2353,.T.);
#3243=ORIENTED_EDGE('',*,*,#2354,.T.);
#3244=ORIENTED_EDGE('',*,*,#2355,.T.);
#3245=ORIENTED_EDGE('',*,*,#2356,.T.);
#3246=ORIENTED_EDGE('',*,*,#2357,.F.);
#3247=ORIENTED_EDGE('',*,*,#2358,.T.);
#3248=ORIENTED_EDGE('',*,*,#2359,.T.);
#3249=ORIENTED_EDGE('',*,*,#2360,.T.);
#3250=ORIENTED_EDGE('',*,*,#2361,.T.);
#3251=ORIENTED_EDGE('',*,*,#2362,.T.);
#3252=ORIENTED_EDGE('',*,*,#2363,.T.);
#3253=ORIENTED_EDGE('',*,*,#2364,.T.);
#3254=ORIENTED_EDGE('',*,*,#2365,.F.);
#3255=ORIENTED_EDGE('',*,*,#2366,.T.);
#3256=ORIENTED_EDGE('',*,*,#2367,.T.);
#3257=ORIENTED_EDGE('',*,*,#2368,.T.);
#3258=ORIENTED_EDGE('',*,*,#2369,.T.);
#3259=ORIENTED_EDGE('',*,*,#2334,.F.);
#3260=ORIENTED_EDGE('',*,*,#2370,.T.);
#3261=ORIENTED_EDGE('',*,*,#2342,.T.);
#3262=ORIENTED_EDGE('',*,*,#2371,.T.);
#3263=ORIENTED_EDGE('',*,*,#2372,.T.);
#3264=ORIENTED_EDGE('',*,*,#2373,.T.);
#3265=ORIENTED_EDGE('',*,*,#2374,.F.);
#3266=ORIENTED_EDGE('',*,*,#2375,.T.);
#3267=ORIENTED_EDGE('',*,*,#2376,.T.);
#3268=ORIENTED_EDGE('',*,*,#2377,.T.);
#3269=ORIENTED_EDGE('',*,*,#2378,.T.);
#3270=ORIENTED_EDGE('',*,*,#2379,.T.);
#3271=ORIENTED_EDGE('',*,*,#2357,.T.);
#3272=ORIENTED_EDGE('',*,*,#2380,.T.);
#3273=ORIENTED_EDGE('',*,*,#2381,.T.);
#3274=ORIENTED_EDGE('',*,*,#2382,.T.);
#3275=ORIENTED_EDGE('',*,*,#2383,.T.);
#3276=ORIENTED_EDGE('',*,*,#2384,.T.);
#3277=ORIENTED_EDGE('',*,*,#2385,.F.);
#3278=ORIENTED_EDGE('',*,*,#2386,.T.);
#3279=ORIENTED_EDGE('',*,*,#2359,.F.);
#3280=ORIENTED_EDGE('',*,*,#2387,.T.);
#3281=ORIENTED_EDGE('',*,*,#2388,.F.);
#3282=ORIENTED_EDGE('',*,*,#2389,.T.);
#3283=ORIENTED_EDGE('',*,*,#2350,.T.);
#3284=ORIENTED_EDGE('',*,*,#2390,.T.);
#3285=ORIENTED_EDGE('',*,*,#2365,.T.);
#3286=ORIENTED_EDGE('',*,*,#2391,.T.);
#3287=ORIENTED_EDGE('',*,*,#2392,.T.);
#3288=ORIENTED_EDGE('',*,*,#2393,.T.);
#3289=ORIENTED_EDGE('',*,*,#2363,.F.);
#3290=ORIENTED_EDGE('',*,*,#2394,.T.);
#3291=ORIENTED_EDGE('',*,*,#2352,.F.);
#3292=ORIENTED_EDGE('',*,*,#2395,.T.);
#3293=ORIENTED_EDGE('',*,*,#2396,.F.);
#3294=ORIENTED_EDGE('',*,*,#2397,.T.);
#3295=ORIENTED_EDGE('',*,*,#2374,.T.);
#3296=ORIENTED_EDGE('',*,*,#2398,.T.);
#3297=ORIENTED_EDGE('',*,*,#2399,.T.);
#3298=ORIENTED_EDGE('',*,*,#2400,.T.);
#3299=ORIENTED_EDGE('',*,*,#2401,.T.);
#3300=ORIENTED_EDGE('',*,*,#2402,.T.);
#3301=ORIENTED_EDGE('',*,*,#2403,.F.);
#3302=ORIENTED_EDGE('',*,*,#2404,.T.);
#3303=ORIENTED_EDGE('',*,*,#2376,.F.);
#3304=ORIENTED_EDGE('',*,*,#2405,.T.);
#3305=ORIENTED_EDGE('',*,*,#2406,.F.);
#3306=ORIENTED_EDGE('',*,*,#2407,.T.);
#3307=ORIENTED_EDGE('',*,*,#2408,.F.);
#3308=ORIENTED_EDGE('',*,*,#2367,.F.);
#3309=ORIENTED_EDGE('',*,*,#2409,.T.);
#3310=ORIENTED_EDGE('',*,*,#2410,.T.);
#3311=ORIENTED_EDGE('',*,*,#2411,.T.);
#3312=ORIENTED_EDGE('',*,*,#2412,.F.);
#3313=ORIENTED_EDGE('',*,*,#2413,.T.);
#3314=ORIENTED_EDGE('',*,*,#2414,.T.);
#3315=ORIENTED_EDGE('',*,*,#2415,.T.);
#3316=ORIENTED_EDGE('',*,*,#2378,.F.);
#3317=ORIENTED_EDGE('',*,*,#2416,.T.);
#3318=ORIENTED_EDGE('',*,*,#2417,.T.);
#3319=ORIENTED_EDGE('',*,*,#2418,.T.);
#3320=ORIENTED_EDGE('',*,*,#2372,.F.);
#3321=ORIENTED_EDGE('',*,*,#2419,.T.);
#3322=ORIENTED_EDGE('',*,*,#2420,.T.);
#3323=ORIENTED_EDGE('',*,*,#2421,.T.);
#3324=ORIENTED_EDGE('',*,*,#2368,.F.);
#3325=ORIENTED_EDGE('',*,*,#2408,.T.);
#3326=ORIENTED_EDGE('',*,*,#2354,.F.);
#3327=ORIENTED_EDGE('',*,*,#2422,.T.);
#3328=ORIENTED_EDGE('',*,*,#2420,.F.);
#3329=ORIENTED_EDGE('',*,*,#2423,.T.);
#3330=ORIENTED_EDGE('',*,*,#2348,.F.);
#3331=ORIENTED_EDGE('',*,*,#2424,.T.);
#3332=ORIENTED_EDGE('',*,*,#2417,.F.);
#3333=ORIENTED_EDGE('',*,*,#2425,.T.);
#3334=ORIENTED_EDGE('',*,*,#2426,.F.);
#3335=ORIENTED_EDGE('',*,*,#2427,.T.);
#3336=ORIENTED_EDGE('',*,*,#2414,.F.);
#3337=ORIENTED_EDGE('',*,*,#2428,.T.);
#3338=ORIENTED_EDGE('',*,*,#2361,.F.);
#3339=ORIENTED_EDGE('',*,*,#2429,.T.);
#3340=ORIENTED_EDGE('',*,*,#2410,.F.);
#3341=ORIENTED_EDGE('',*,*,#2430,.T.);
#3342=ORIENTED_EDGE('',*,*,#2355,.F.);
#3343=ORIENTED_EDGE('',*,*,#2403,.T.);
#3344=ORIENTED_EDGE('',*,*,#2431,.T.);
#3345=ORIENTED_EDGE('',*,*,#2399,.F.);
#3346=ORIENTED_EDGE('',*,*,#2432,.T.);
#3347=ORIENTED_EDGE('',*,*,#2426,.T.);
#3348=ORIENTED_EDGE('',*,*,#2433,.T.);
#3349=ORIENTED_EDGE('',*,*,#2385,.T.);
#3350=ORIENTED_EDGE('',*,*,#2434,.T.);
#3351=ORIENTED_EDGE('',*,*,#2381,.F.);
#3352=ORIENTED_EDGE('',*,*,#2435,.T.);
#3353=ORIENTED_EDGE('',*,*,#2412,.T.);
#3354=ORIENTED_EDGE('',*,*,#2436,.T.);
#3355=ORIENTED_EDGE('',*,*,#2437,.T.);
#3356=ORIENTED_EDGE('',*,*,#2438,.T.);
#3357=ORIENTED_EDGE('',*,*,#2439,.T.);
#3358=ORIENTED_EDGE('',*,*,#2396,.T.);
#3359=ORIENTED_EDGE('',*,*,#2440,.T.);
#3360=ORIENTED_EDGE('',*,*,#2441,.T.);
#3361=ORIENTED_EDGE('',*,*,#2442,.F.);
#3362=ORIENTED_EDGE('',*,*,#2441,.F.);
#3363=ORIENTED_EDGE('',*,*,#2443,.T.);
#3364=ORIENTED_EDGE('',*,*,#2392,.F.);
#3365=ORIENTED_EDGE('',*,*,#2444,.T.);
#3366=ORIENTED_EDGE('',*,*,#2438,.F.);
#3367=ORIENTED_EDGE('',*,*,#2445,.T.);
#3368=ORIENTED_EDGE('',*,*,#2383,.F.);
#3369=ORIENTED_EDGE('',*,*,#2446,.T.);
#3370=ORIENTED_EDGE('',*,*,#2388,.T.);
#3371=ORIENTED_EDGE('',*,*,#2447,.T.);
#3372=ORIENTED_EDGE('',*,*,#2406,.T.);
#3373=ORIENTED_EDGE('',*,*,#2448,.T.);
#3374=ORIENTED_EDGE('',*,*,#2401,.F.);
#3375=ORIENTED_EDGE('',*,*,#2449,.T.);
#3376=ORIENTED_EDGE('',*,*,#2338,.F.);
#3377=ORIENTED_EDGE('',*,*,#2450,.T.);
#3378=ORIENTED_EDGE('',*,*,#2344,.T.);
#3379=ORIENTED_EDGE('',*,*,#2442,.T.);
#3380=ORIENTED_EDGE('',*,*,#2451,.T.);
#3381=ORIENTED_EDGE('',*,*,#2452,.T.);
#3382=ORIENTED_EDGE('',*,*,#2453,.T.);
#3383=ORIENTED_EDGE('',*,*,#2454,.T.);
#3384=ORIENTED_EDGE('',*,*,#2437,.F.);
#3385=ORIENTED_EDGE('',*,*,#2455,.F.);
#3386=ORIENTED_EDGE('',*,*,#2456,.F.);
#3387=ORIENTED_EDGE('',*,*,#2457,.F.);
#3388=ORIENTED_EDGE('',*,*,#2458,.F.);
#3389=ORIENTED_EDGE('',*,*,#2456,.T.);
#3390=ORIENTED_EDGE('',*,*,#2459,.F.);
#3391=ORIENTED_EDGE('',*,*,#2451,.F.);
#3392=ORIENTED_EDGE('',*,*,#2460,.T.);
#3393=ORIENTED_EDGE('',*,*,#2457,.T.);
#3394=ORIENTED_EDGE('',*,*,#2460,.F.);
#3395=ORIENTED_EDGE('',*,*,#2454,.F.);
#3396=ORIENTED_EDGE('',*,*,#2461,.T.);
#3397=ORIENTED_EDGE('',*,*,#2458,.T.);
#3398=ORIENTED_EDGE('',*,*,#2461,.F.);
#3399=ORIENTED_EDGE('',*,*,#2453,.F.);
#3400=ORIENTED_EDGE('',*,*,#2462,.T.);
#3401=ORIENTED_EDGE('',*,*,#2455,.T.);
#3402=ORIENTED_EDGE('',*,*,#2462,.F.);
#3403=ORIENTED_EDGE('',*,*,#2452,.F.);
#3404=ORIENTED_EDGE('',*,*,#2459,.T.);
#3405=ORIENTED_EDGE('',*,*,#2395,.F.);
#3406=ORIENTED_EDGE('',*,*,#2351,.F.);
#3407=ORIENTED_EDGE('',*,*,#2393,.F.);
#3408=ORIENTED_EDGE('',*,*,#2443,.F.);
#3409=ORIENTED_EDGE('',*,*,#2440,.F.);
#3410=ORIENTED_EDGE('',*,*,#2343,.F.);
#3411=ORIENTED_EDGE('',*,*,#2370,.F.);
#3412=ORIENTED_EDGE('',*,*,#2339,.F.);
#3413=ORIENTED_EDGE('',*,*,#2449,.F.);
#3414=ORIENTED_EDGE('',*,*,#2391,.F.);
#3415=ORIENTED_EDGE('',*,*,#2364,.F.);
#3416=ORIENTED_EDGE('',*,*,#2397,.F.);
#3417=ORIENTED_EDGE('',*,*,#2439,.F.);
#3418=ORIENTED_EDGE('',*,*,#2444,.F.);
#3419=ORIENTED_EDGE('',*,*,#2337,.F.);
#3420=ORIENTED_EDGE('',*,*,#2346,.F.);
#3421=ORIENTED_EDGE('',*,*,#2345,.F.);
#3422=ORIENTED_EDGE('',*,*,#2450,.F.);
#3423=ORIENTED_EDGE('',*,*,#2400,.F.);
#3424=ORIENTED_EDGE('',*,*,#2431,.F.);
#3425=ORIENTED_EDGE('',*,*,#2407,.F.);
#3426=ORIENTED_EDGE('',*,*,#2447,.F.);
#3427=ORIENTED_EDGE('',*,*,#2387,.F.);
#3428=ORIENTED_EDGE('',*,*,#2358,.F.);
#3429=ORIENTED_EDGE('',*,*,#2384,.F.);
#3430=ORIENTED_EDGE('',*,*,#2445,.F.);
#3431=ORIENTED_EDGE('',*,*,#2382,.F.);
#3432=ORIENTED_EDGE('',*,*,#2434,.F.);
#3433=ORIENTED_EDGE('',*,*,#2389,.F.);
#3434=ORIENTED_EDGE('',*,*,#2446,.F.);
#3435=ORIENTED_EDGE('',*,*,#2405,.F.);
#3436=ORIENTED_EDGE('',*,*,#2375,.F.);
#3437=ORIENTED_EDGE('',*,*,#2402,.F.);
#3438=ORIENTED_EDGE('',*,*,#2448,.F.);
#3439=ORIENTED_EDGE('',*,*,#2347,.F.);
#3440=ORIENTED_EDGE('',*,*,#2335,.F.);
#3441=ORIENTED_EDGE('',*,*,#2373,.F.);
#3442=ORIENTED_EDGE('',*,*,#2418,.F.);
#3443=ORIENTED_EDGE('',*,*,#2424,.F.);
#3444=ORIENTED_EDGE('',*,*,#2349,.F.);
#3445=ORIENTED_EDGE('',*,*,#2423,.F.);
#3446=ORIENTED_EDGE('',*,*,#2419,.F.);
#3447=ORIENTED_EDGE('',*,*,#2371,.F.);
#3448=ORIENTED_EDGE('',*,*,#2341,.F.);
#3449=ORIENTED_EDGE('',*,*,#2432,.F.);
#3450=ORIENTED_EDGE('',*,*,#2398,.F.);
#3451=ORIENTED_EDGE('',*,*,#2379,.F.);
#3452=ORIENTED_EDGE('',*,*,#2415,.F.);
#3453=ORIENTED_EDGE('',*,*,#2427,.F.);
#3454=ORIENTED_EDGE('',*,*,#2433,.F.);
#3455=ORIENTED_EDGE('',*,*,#2425,.F.);
#3456=ORIENTED_EDGE('',*,*,#2416,.F.);
#3457=ORIENTED_EDGE('',*,*,#2377,.F.);
#3458=ORIENTED_EDGE('',*,*,#2404,.F.);
#3459=ORIENTED_EDGE('',*,*,#2369,.F.);
#3460=ORIENTED_EDGE('',*,*,#2421,.F.);
#3461=ORIENTED_EDGE('',*,*,#2422,.F.);
#3462=ORIENTED_EDGE('',*,*,#2353,.F.);
#3463=ORIENTED_EDGE('',*,*,#2394,.F.);
#3464=ORIENTED_EDGE('',*,*,#2366,.F.);
#3465=ORIENTED_EDGE('',*,*,#2390,.F.);
#3466=ORIENTED_EDGE('',*,*,#2356,.F.);
#3467=ORIENTED_EDGE('',*,*,#2430,.F.);
#3468=ORIENTED_EDGE('',*,*,#2409,.F.);
#3469=ORIENTED_EDGE('',*,*,#2436,.F.);
#3470=ORIENTED_EDGE('',*,*,#2411,.F.);
#3471=ORIENTED_EDGE('',*,*,#2429,.F.);
#3472=ORIENTED_EDGE('',*,*,#2360,.F.);
#3473=ORIENTED_EDGE('',*,*,#2386,.F.);
#3474=ORIENTED_EDGE('',*,*,#2435,.F.);
#3475=ORIENTED_EDGE('',*,*,#2380,.F.);
#3476=ORIENTED_EDGE('',*,*,#2362,.F.);
#3477=ORIENTED_EDGE('',*,*,#2428,.F.);
#3478=ORIENTED_EDGE('',*,*,#2413,.F.);
#3649=TOROIDAL_SURFACE('',#4355,79.,10.);
#3650=TOROIDAL_SURFACE('',#4386,18.,2.);
#3651=TOROIDAL_SURFACE('',#4387,18.,2.);
#3652=TOROIDAL_SURFACE('',#4388,18.,2.);
#3653=TOROIDAL_SURFACE('',#4389,18.,2.);
#3654=TOROIDAL_SURFACE('',#4390,18.,2.);
#3655=TOROIDAL_SURFACE('',#4391,18.,2.);
#3656=TOROIDAL_SURFACE('',#4392,18.,2.);
#3657=TOROIDAL_SURFACE('',#4393,18.,2.);
#3804=ADVANCED_FACE('',(#956),#332,.T.);
#3805=ADVANCED_FACE('',(#957),#333,.F.);
#3806=ADVANCED_FACE('',(#958),#334,.F.);
#3807=ADVANCED_FACE('',(#959),#335,.F.);
#3808=ADVANCED_FACE('',(#960),#336,.F.);
#3809=ADVANCED_FACE('',(#961),#337,.F.);
#3810=ADVANCED_FACE('',(#962),#338,.F.);
#3811=ADVANCED_FACE('',(#963),#339,.F.);
#3812=ADVANCED_FACE('',(#964),#340,.T.);
#3813=ADVANCED_FACE('',(#965),#341,.F.);
#3814=ADVANCED_FACE('',(#966),#342,.T.);
#3815=ADVANCED_FACE('',(#967),#343,.F.);
#3816=ADVANCED_FACE('',(#968),#344,.T.);
#3817=ADVANCED_FACE('',(#969),#345,.F.);
#3818=ADVANCED_FACE('',(#970),#3649,.T.);
#3819=ADVANCED_FACE('',(#971),#346,.F.);
#3820=ADVANCED_FACE('',(#972),#347,.F.);
#3821=ADVANCED_FACE('',(#973,#260,#261,#262),#807,.T.);
#3822=ADVANCED_FACE('',(#974,#263),#348,.T.);
#3823=ADVANCED_FACE('',(#975,#264),#349,.F.);
#3824=ADVANCED_FACE('',(#976),#350,.F.);
#3825=ADVANCED_FACE('',(#977),#351,.F.);
#3826=ADVANCED_FACE('',(#978),#352,.F.);
#3827=ADVANCED_FACE('',(#979),#353,.F.);
#3828=ADVANCED_FACE('',(#980),#3650,.F.);
#3829=ADVANCED_FACE('',(#981),#3651,.F.);
#3830=ADVANCED_FACE('',(#982),#3652,.F.);
#3831=ADVANCED_FACE('',(#983),#3653,.F.);
#3832=ADVANCED_FACE('',(#984),#3654,.F.);
#3833=ADVANCED_FACE('',(#985),#3655,.F.);
#3834=ADVANCED_FACE('',(#986),#3656,.F.);
#3835=ADVANCED_FACE('',(#987),#3657,.F.);
#3836=ADVANCED_FACE('',(#988),#67,.F.);
#3837=ADVANCED_FACE('',(#989),#68,.F.);
#3838=ADVANCED_FACE('',(#990),#69,.F.);
#3839=ADVANCED_FACE('',(#991),#70,.F.);
#3840=ADVANCED_FACE('',(#992),#71,.F.);
#3841=ADVANCED_FACE('',(#993),#72,.F.);
#3842=ADVANCED_FACE('',(#994),#73,.F.);
#3843=ADVANCED_FACE('',(#995),#74,.F.);
#3889=CLOSED_SHELL('',(#3804,#3805,#3806,#3807,#3808,#3809,#3810,#3811,
#3812,#3813,#3814,#3815,#3816,#3817,#3818,#3819,#3820,#3821,#3822,#3823,
#3824,#3825,#3826,#3827,#3828,#3829,#3830,#3831,#3832,#3833,#3834,#3835,
#3836,#3837,#3838,#3839,#3840,#3841,#3842,#3843));
#4326=AXIS2_PLACEMENT_3D('',#7168,#5226,#5227);
#4327=AXIS2_PLACEMENT_3D('',#7169,#5228,#5229);
#4328=AXIS2_PLACEMENT_3D('',#7287,#5233,#5234);
#4329=AXIS2_PLACEMENT_3D('',#7408,#5238,#5239);
#4330=AXIS2_PLACEMENT_3D('',#7409,#5240,#5241);
#4331=AXIS2_PLACEMENT_3D('',#7424,#5242,#5243);
#4332=AXIS2_PLACEMENT_3D('',#7437,#5244,#5245);
#4333=AXIS2_PLACEMENT_3D('',#7442,#5247,#5248);
#4334=AXIS2_PLACEMENT_3D('',#7459,#5250,#5251);
#4335=AXIS2_PLACEMENT_3D('',#7461,#5252,#5253);
#4336=AXIS2_PLACEMENT_3D('',#7474,#5254,#5255);
#4337=AXIS2_PLACEMENT_3D('',#7479,#5257,#5258);
#4338=AXIS2_PLACEMENT_3D('',#7496,#5260,#5261);
#4339=AXIS2_PLACEMENT_3D('',#7509,#5262,#5263);
#4340=AXIS2_PLACEMENT_3D('',#7514,#5265,#5266);
#4341=AXIS2_PLACEMENT_3D('',#7531,#5268,#5269);
#4342=AXIS2_PLACEMENT_3D('',#7533,#5270,#5271);
#4343=AXIS2_PLACEMENT_3D('',#7546,#5272,#5273);
#4344=AXIS2_PLACEMENT_3D('',#7547,#5274,#5275);
#4345=AXIS2_PLACEMENT_3D('',#7562,#5276,#5277);
#4346=AXIS2_PLACEMENT_3D('',#7575,#5278,#5279);
#4347=AXIS2_PLACEMENT_3D('',#7580,#5281,#5282);
#4348=AXIS2_PLACEMENT_3D('',#7597,#5284,#5285);
#4349=AXIS2_PLACEMENT_3D('',#7610,#5286,#5287);
#4350=AXIS2_PLACEMENT_3D('',#7725,#5290,#5291);
#4351=AXIS2_PLACEMENT_3D('',#7834,#5294,#5295);
#4352=AXIS2_PLACEMENT_3D('',#7943,#5297,#5298);
#4353=AXIS2_PLACEMENT_3D('',#8055,#5300,#5301);
#4354=AXIS2_PLACEMENT_3D('',#8173,#5304,#5305);
#4355=AXIS2_PLACEMENT_3D('',#8285,#5308,#5309);
#4356=AXIS2_PLACEMENT_3D('',#8286,#5310,#5311);
#4357=AXIS2_PLACEMENT_3D('',#8299,#5312,#5313);
#4358=AXIS2_PLACEMENT_3D('',#8354,#5314,#5315);
#4359=AXIS2_PLACEMENT_3D('',#8368,#5316,#5317);
#4360=AXIS2_PLACEMENT_3D('',#8436,#5318,#5319);
#4361=AXIS2_PLACEMENT_3D('',#8540,#5320,#5321);
#4362=AXIS2_PLACEMENT_3D('',#8747,#5322,#5323);
#4363=AXIS2_PLACEMENT_3D('',#8869,#5324,#5325);
#4364=AXIS2_PLACEMENT_3D('',#8870,#5326,#5327);
#4365=AXIS2_PLACEMENT_3D('',#8895,#5328,#5329);
#4366=AXIS2_PLACEMENT_3D('',#8896,#5330,#5331);
#4367=AXIS2_PLACEMENT_3D('',#8921,#5332,#5333);
#4368=AXIS2_PLACEMENT_3D('',#8923,#5334,#5335);
#4369=AXIS2_PLACEMENT_3D('',#8926,#5337,#5338);
#4370=AXIS2_PLACEMENT_3D('',#8928,#5339,#5340);
#4371=AXIS2_PLACEMENT_3D('',#8931,#5342,#5343);
#4372=AXIS2_PLACEMENT_3D('',#8932,#5344,#5345);
#4373=AXIS2_PLACEMENT_3D('',#8933,#5346,#5347);
#4374=AXIS2_PLACEMENT_3D('',#8934,#5348,#5349);
#4375=AXIS2_PLACEMENT_3D('',#8935,#5350,#5351);
#4376=AXIS2_PLACEMENT_3D('',#8936,#5352,#5353);
#4377=AXIS2_PLACEMENT_3D('',#8937,#5354,#5355);
#4378=AXIS2_PLACEMENT_3D('',#8938,#5356,#5357);
#4379=AXIS2_PLACEMENT_3D('',#8939,#5358,#5359);
#4380=AXIS2_PLACEMENT_3D('',#8940,#5360,#5361);
#4381=AXIS2_PLACEMENT_3D('',#8949,#5366,#5367);
#4382=AXIS2_PLACEMENT_3D('',#8958,#5372,#5373);
#4383=AXIS2_PLACEMENT_3D('',#8961,#5376,#5377);
#4384=AXIS2_PLACEMENT_3D('',#8963,#5379,#5380);
#4385=AXIS2_PLACEMENT_3D('',#8965,#5382,#5383);
#4386=AXIS2_PLACEMENT_3D('',#8966,#5384,#5385);
#4387=AXIS2_PLACEMENT_3D('',#8967,#5386,#5387);
#4388=AXIS2_PLACEMENT_3D('',#8968,#5388,#5389);
#4389=AXIS2_PLACEMENT_3D('',#8969,#5390,#5391);
#4390=AXIS2_PLACEMENT_3D('',#8970,#5392,#5393);
#4391=AXIS2_PLACEMENT_3D('',#8971,#5394,#5395);
#4392=AXIS2_PLACEMENT_3D('',#8972,#5396,#5397);
#4393=AXIS2_PLACEMENT_3D('',#8973,#5398,#5399);
#5226=DIRECTION('axis',(0.,0.,1.));
#5227=DIRECTION('refdir',(1.,0.,0.));
#5228=DIRECTION('center_axis',(0.,0.,1.));
#5229=DIRECTION('ref_axis',(1.,0.,0.));
#5230=DIRECTION('',(4.33942623640377E-17,-1.,0.));
#5231=DIRECTION('',(0.,1.,0.));
#5232=DIRECTION('',(-1.,0.,0.));
#5233=DIRECTION('center_axis',(0.,0.,1.));
#5234=DIRECTION('ref_axis',(1.,0.,0.));
#5235=DIRECTION('',(0.,1.,0.));
#5236=DIRECTION('',(4.33942623640377E-17,-1.,0.));
#5237=DIRECTION('',(-1.,0.,0.));
#5238=DIRECTION('center_axis',(-1.,0.,0.));
#5239=DIRECTION('ref_axis',(0.,0.,1.));
#5240=DIRECTION('center_axis',(-1.,0.,0.));
#5241=DIRECTION('ref_axis',(0.,0.,1.));
#5242=DIRECTION('center_axis',(1.,0.,0.));
#5243=DIRECTION('ref_axis',(0.,0.,-1.));
#5244=DIRECTION('center_axis',(-1.,0.,0.));
#5245=DIRECTION('ref_axis',(0.,0.,1.));
#5246=DIRECTION('',(0.,-3.49323812030503E-15,-1.));
#5247=DIRECTION('center_axis',(-1.,0.,0.));
#5248=DIRECTION('ref_axis',(0.,0.,1.));
#5249=DIRECTION('',(0.,-3.49323812030503E-15,-1.));
#5250=DIRECTION('center_axis',(1.,0.,0.));
#5251=DIRECTION('ref_axis',(0.,0.,-1.));
#5252=DIRECTION('center_axis',(1.,0.,0.));
#5253=DIRECTION('ref_axis',(0.,0.,-1.));
#5254=DIRECTION('center_axis',(-1.,0.,0.));
#5255=DIRECTION('ref_axis',(0.,0.,1.));
#5256=DIRECTION('',(0.,1.,0.));
#5257=DIRECTION('center_axis',(-1.,0.,0.));
#5258=DIRECTION('ref_axis',(0.,0.,1.));
#5259=DIRECTION('',(0.,1.,0.));
#5260=DIRECTION('center_axis',(1.,0.,0.));
#5261=DIRECTION('ref_axis',(0.,0.,-1.));
#5262=DIRECTION('center_axis',(1.,5.88949328263731E-17,0.));
#5263=DIRECTION('ref_axis',(0.,0.,-1.));
#5264=DIRECTION('',(6.50913935460565E-17,3.49323812030503E-15,1.));
#5265=DIRECTION('center_axis',(1.,5.88949328263731E-17,0.));
#5266=DIRECTION('ref_axis',(-5.88949328263731E-17,1.,0.));
#5267=DIRECTION('',(6.50913935460565E-17,3.49323812030503E-15,1.));
#5268=DIRECTION('center_axis',(-1.,2.05630558915701E-31,5.88949328263731E-17));
#5269=DIRECTION('ref_axis',(5.88949328263731E-17,0.,1.));
#5270=DIRECTION('center_axis',(-1.,2.05630558915701E-31,5.88949328263731E-17));
#5271=DIRECTION('ref_axis',(5.88949328263731E-17,0.,1.));
#5272=DIRECTION('center_axis',(1.,5.88949328263731E-17,0.));
#5273=DIRECTION('ref_axis',(0.,0.,-1.));
#5274=DIRECTION('center_axis',(1.,5.88949328263731E-17,0.));
#5275=DIRECTION('ref_axis',(-5.88949328263731E-17,1.,0.));
#5276=DIRECTION('center_axis',(-1.,-5.88949328263731E-17,0.));
#5277=DIRECTION('ref_axis',(5.88949328263731E-17,-1.,0.));
#5278=DIRECTION('center_axis',(1.,5.88949328263731E-17,0.));
#5279=DIRECTION('ref_axis',(0.,0.,-1.));
#5280=DIRECTION('',(4.33942623640377E-17,3.49323812030503E-15,1.));
#5281=DIRECTION('center_axis',(1.,5.88949328263731E-17,0.));
#5282=DIRECTION('ref_axis',(-5.88949328263731E-17,1.,0.));
#5283=DIRECTION('',(4.33942623640377E-17,3.49323812030503E-15,1.));
#5284=DIRECTION('center_axis',(-1.,2.05630558915701E-31,5.88949328263731E-17));
#5285=DIRECTION('ref_axis',(5.88949328263731E-17,0.,1.));
#5286=DIRECTION('center_axis',(0.,0.,1.));
#5287=DIRECTION('ref_axis',(1.,0.,0.));
#5288=DIRECTION('',(6.50913935460565E-17,-1.,0.));
#5289=DIRECTION('',(-1.,0.,0.));
#5290=DIRECTION('center_axis',(0.,0.,1.));
#5291=DIRECTION('ref_axis',(1.,0.,0.));
#5292=DIRECTION('',(6.50913935460565E-17,-1.,0.));
#5293=DIRECTION('',(-1.,0.,0.));
#5294=DIRECTION('center_axis',(0.,1.,-3.49148133884313E-15));
#5295=DIRECTION('ref_axis',(0.,3.49148133884313E-15,1.));
#5296=DIRECTION('',(-1.,0.,0.));
#5297=DIRECTION('center_axis',(0.,1.,-3.49148133884313E-15));
#5298=DIRECTION('ref_axis',(0.,3.49148133884313E-15,1.));
#5299=DIRECTION('',(-1.,0.,0.));
#5300=DIRECTION('center_axis',(0.,1.,-3.49148133884313E-15));
#5301=DIRECTION('ref_axis',(0.,3.49148133884313E-15,1.));
#5302=DIRECTION('',(0.,-3.49323812030503E-15,-1.));
#5303=DIRECTION('',(-1.,0.,0.));
#5304=DIRECTION('center_axis',(0.,1.,-3.49148133884313E-15));
#5305=DIRECTION('ref_axis',(0.,3.49148133884313E-15,1.));
#5306=DIRECTION('',(0.,-3.49323812030503E-15,-1.));
#5307=DIRECTION('',(-1.,0.,0.));
#5308=DIRECTION('center_axis',(-1.,0.,0.));
#5309=DIRECTION('ref_axis',(0.,0.,1.));
#5310=DIRECTION('center_axis',(0.,-1.,1.22464679914735E-16));
#5311=DIRECTION('ref_axis',(0.,-1.22464679914735E-16,-1.));
#5312=DIRECTION('center_axis',(1.,0.,0.));
#5313=DIRECTION('ref_axis',(0.,0.,1.));
#5314=DIRECTION('center_axis',(-1.,-5.88949328263731E-17,0.));
#5315=DIRECTION('ref_axis',(5.88949328263731E-17,-1.,0.));
#5316=DIRECTION('center_axis',(1.,0.,0.));
#5317=DIRECTION('ref_axis',(0.,0.,1.));
#5318=DIRECTION('center_axis',(1.,0.,0.));
#5319=DIRECTION('ref_axis',(0.,0.,1.));
#5320=DIRECTION('center_axis',(1.,0.,0.));
#5321=DIRECTION('ref_axis',(0.,0.,1.));
#5322=DIRECTION('center_axis',(1.,0.,0.));
#5323=DIRECTION('ref_axis',(0.,0.,-1.));
#5324=DIRECTION('center_axis',(-1.,0.,0.));
#5325=DIRECTION('ref_axis',(0.,0.,1.));
#5326=DIRECTION('center_axis',(-1.,0.,0.));
#5327=DIRECTION('ref_axis',(0.,0.,1.));
#5328=DIRECTION('center_axis',(1.,5.88949328263731E-17,0.));
#5329=DIRECTION('ref_axis',(0.,0.,-1.));
#5330=DIRECTION('center_axis',(1.,5.88949328263731E-17,0.));
#5331=DIRECTION('ref_axis',(-5.88949328263731E-17,1.,0.));
#5332=DIRECTION('center_axis',(-1.,0.,0.));
#5333=DIRECTION('ref_axis',(0.,0.,1.));
#5334=DIRECTION('center_axis',(1.,0.,0.));
#5335=DIRECTION('ref_axis',(0.,0.,-1.));
#5336=DIRECTION('',(1.,0.,0.));
#5337=DIRECTION('center_axis',(1.,5.88949328263731E-17,0.));
#5338=DIRECTION('ref_axis',(-5.88949328263731E-17,1.,0.));
#5339=DIRECTION('center_axis',(-1.,0.,0.));
#5340=DIRECTION('ref_axis',(0.,0.,1.));
#5341=DIRECTION('',(1.,0.,0.));
#5342=DIRECTION('center_axis',(1.,0.,0.));
#5343=DIRECTION('ref_axis',(0.,0.,-1.));
#5344=DIRECTION('center_axis',(-1.,0.,0.));
#5345=DIRECTION('ref_axis',(0.,0.,1.));
#5346=DIRECTION('center_axis',(1.,5.88949328263731E-17,0.));
#5347=DIRECTION('ref_axis',(-5.88949328263731E-17,1.,0.));
#5348=DIRECTION('center_axis',(-1.,0.,0.));
#5349=DIRECTION('ref_axis',(0.,0.,1.));
#5350=DIRECTION('center_axis',(1.,5.88949328263731E-17,0.));
#5351=DIRECTION('ref_axis',(-5.88949328263731E-17,1.,0.));
#5352=DIRECTION('center_axis',(-1.,0.,0.));
#5353=DIRECTION('ref_axis',(0.,0.,1.));
#5354=DIRECTION('center_axis',(1.,5.88949328263731E-17,0.));
#5355=DIRECTION('ref_axis',(-5.88949328263731E-17,1.,0.));
#5356=DIRECTION('center_axis',(1.,5.88949328263731E-17,0.));
#5357=DIRECTION('ref_axis',(-5.88949328263731E-17,1.,0.));
#5358=DIRECTION('center_axis',(-1.,0.,0.));
#5359=DIRECTION('ref_axis',(0.,0.,1.));
#5360=DIRECTION('center_axis',(1.,0.,0.));
#5361=DIRECTION('ref_axis',(0.,0.,-1.));
#5362=DIRECTION('',(0.,1.,-1.85037170770859E-16));
#5363=DIRECTION('',(0.,0.,-1.));
#5364=DIRECTION('',(0.,-1.,1.85037170770859E-16));
#5365=DIRECTION('',(0.,0.,1.));
#5366=DIRECTION('center_axis',(1.,0.,0.));
#5367=DIRECTION('ref_axis',(0.,0.,-1.));
#5368=DIRECTION('',(0.,0.,-1.));
#5369=DIRECTION('',(0.,1.,-1.85037170770859E-16));
#5370=DIRECTION('',(0.,0.,1.));
#5371=DIRECTION('',(0.,-1.,1.85037170770859E-16));
#5372=DIRECTION('center_axis',(0.,1.44560289664734E-16,1.));
#5373=DIRECTION('ref_axis',(1.,0.,0.));
#5374=DIRECTION('',(-1.,0.,0.));
#5375=DIRECTION('',(-1.,0.,0.));
#5376=DIRECTION('center_axis',(0.,-1.,0.));
#5377=DIRECTION('ref_axis',(0.,0.,-1.));
#5378=DIRECTION('',(-1.,0.,0.));
#5379=DIRECTION('center_axis',(0.,-1.44560289664734E-16,-1.));
#5380=DIRECTION('ref_axis',(-1.,0.,0.));
#5381=DIRECTION('',(-1.,0.,0.));
#5382=DIRECTION('center_axis',(0.,1.,0.));
#5383=DIRECTION('ref_axis',(0.,0.,1.));
#5384=DIRECTION('center_axis',(-1.,0.,0.));
#5385=DIRECTION('ref_axis',(0.,-3.67517835871524E-15,-1.));
#5386=DIRECTION('center_axis',(1.,5.88949328263731E-17,0.));
#5387=DIRECTION('ref_axis',(0.,0.,-1.));
#5388=DIRECTION('center_axis',(1.,5.88949328263731E-17,0.));
#5389=DIRECTION('ref_axis',(0.,0.,-1.));
#5390=DIRECTION('center_axis',(-1.,0.,0.));
#5391=DIRECTION('ref_axis',(0.,0.,1.));
#5392=DIRECTION('center_axis',(-1.,0.,0.));
#5393=DIRECTION('ref_axis',(0.,0.,1.));
#5394=DIRECTION('center_axis',(-1.,0.,0.));
#5395=DIRECTION('ref_axis',(0.,0.,1.));
#5396=DIRECTION('center_axis',(1.,5.88949328263731E-17,0.));
#5397=DIRECTION('ref_axis',(0.,0.,-1.));
#5398=DIRECTION('center_axis',(1.,5.88949328263731E-17,0.));
#5399=DIRECTION('ref_axis',(0.,3.43024899888577E-15,1.));
#7168=CARTESIAN_POINT('',(0.,0.,0.));
#7169=CARTESIAN_POINT('Origin',(0.,0.,6.));
#7170=CARTESIAN_POINT('',(-5.99999999999999,-16.9705627484771,6.));
#7171=CARTESIAN_POINT('',(-5.99999999999999,-68.1396788547224,6.));
#7172=CARTESIAN_POINT('',(-5.99999999999999,-16.9705627484771,6.));
#7173=CARTESIAN_POINT('',(5.99999617479513,-68.1397016670827,6.00000000000002));
#7174=CARTESIAN_POINT('Ctrl Pts',(-5.99999999999999,-68.1396788547224,6.00000000012849));
#7175=CARTESIAN_POINT('Ctrl Pts',(-5.88220806812114,-68.0712045447482,6.00000000008163));
#7176=CARTESIAN_POINT('Ctrl Pts',(-5.76349611642723,-68.0048909413794,6.00000000005477));
#7177=CARTESIAN_POINT('Ctrl Pts',(-5.64383895277427,-67.9406843861809,6.00000000003867));
#7178=CARTESIAN_POINT('Ctrl Pts',(-5.35720147136636,-67.7868782561497,6.00000000000011));
#7179=CARTESIAN_POINT('Ctrl Pts',(-5.06513993011167,-67.6451640000266,5.99999999998887));
#7180=CARTESIAN_POINT('Ctrl Pts',(-4.76775535283963,-67.5155036880928,6.00000000004808));
#7181=CARTESIAN_POINT('Ctrl Pts',(-4.70882262228595,-67.4898088914871,6.00000000005981));
#7182=CARTESIAN_POINT('Ctrl Pts',(-4.64968086212463,-67.464587446345,6.00000000007612));
#7183=CARTESIAN_POINT('Ctrl Pts',(-4.59033271641865,-67.4398422796416,6.0000000001009));
#7184=CARTESIAN_POINT('Ctrl Pts',(-4.34878747251347,-67.3391301637743,6.00000000020175));
#7185=CARTESIAN_POINT('Ctrl Pts',(-4.10376784428531,-67.2462488735296,6.00000000005394));
#7186=CARTESIAN_POINT('Ctrl Pts',(-3.85528977251545,-67.1613881052392,6.00000000001804));
#7187=CARTESIAN_POINT('Ctrl Pts',(-3.85490034355802,-67.1612551066197,6.00000000001798));
#7188=CARTESIAN_POINT('Ctrl Pts',(-3.8545109061033,-67.1611221277072,6.00000000001793));
#7189=CARTESIAN_POINT('Ctrl Pts',(-3.85412146016043,-67.160989168504,6.00000000001787));
#7190=CARTESIAN_POINT('Ctrl Pts',(-3.60524310476614,-67.0760205908866,5.99999999998215));
#7191=CARTESIAN_POINT('Ctrl Pts',(-3.35289435328196,-66.9991042097109,6.));
#7192=CARTESIAN_POINT('Ctrl Pts',(-3.09960379879075,-66.9308520752212,6.));
#7193=CARTESIAN_POINT('Ctrl Pts',(-3.03719950469825,-66.9140365003897,6.));
#7194=CARTESIAN_POINT('Ctrl Pts',(-2.97470738560379,-66.8977385562704,6.));
#7195=CARTESIAN_POINT('Ctrl Pts',(-2.91216650726521,-66.8819693081272,6.));
#7196=CARTESIAN_POINT('Ctrl Pts',(-2.64202477002678,-66.8138549451454,6.));
#7197=CARTESIAN_POINT('Ctrl Pts',(-2.37097311554184,-66.7556089621424,6.));
#7198=CARTESIAN_POINT('Ctrl Pts',(-2.09860427727656,-66.7069169291021,6.));
#7199=CARTESIAN_POINT('Ctrl Pts',(-2.05141021421883,-66.698479932813,6.));
#7200=CARTESIAN_POINT('Ctrl Pts',(-2.0041766171422,-66.6903296526791,6.));
#7201=CARTESIAN_POINT('Ctrl Pts',(-1.95690138678829,-66.6824642970514,6.));
#7202=CARTESIAN_POINT('Ctrl Pts',(-1.82742310634297,-66.6609225147239,6.));
#7203=CARTESIAN_POINT('Ctrl Pts',(-1.69763250633901,-66.6415181735337,6.));
#7204=CARTESIAN_POINT('Ctrl Pts',(-1.56756922953221,-66.6242591965759,6.));
#7205=CARTESIAN_POINT('Ctrl Pts',(-1.3759989138017,-66.5988384341119,6.));
#7206=CARTESIAN_POINT('Ctrl Pts',(-1.18372985956116,-66.5780591520956,5.99999999999998));
#7207=CARTESIAN_POINT('Ctrl Pts',(-0.990820807203484,-66.5619477872285,
6.00000000000404));
#7208=CARTESIAN_POINT('Ctrl Pts',(-0.667085375757139,-66.5349100738984,
6.00000000001086));
#7209=CARTESIAN_POINT('Ctrl Pts',(-0.341547876894146,-66.5210179927549,
6.00000000002069));
#7210=CARTESIAN_POINT('Ctrl Pts',(-0.0138882729886304,-66.5206865118667,
6.0000000000061));
#7211=CARTESIAN_POINT('Ctrl Pts',(-0.0118363442197238,-66.5206844360076,
6.00000000000601));
#7212=CARTESIAN_POINT('Ctrl Pts',(-0.00978433221009082,-66.5206828919889,
6.00000000000592));
#7213=CARTESIAN_POINT('Ctrl Pts',(-0.00773223806953993,-66.5206818797792,
6.00000000000582));
#7214=CARTESIAN_POINT('Ctrl Pts',(0.223352402590758,-66.5205678956829,5.99999999999557));
#7215=CARTESIAN_POINT('Ctrl Pts',(0.45544978788947,-66.5272104286493,6.));
#7216=CARTESIAN_POINT('Ctrl Pts',(0.686742750504859,-66.5405340810191,6.));
#7217=CARTESIAN_POINT('Ctrl Pts',(0.718187055372043,-66.5423454330911,6.));
#7218=CARTESIAN_POINT('Ctrl Pts',(0.749616505983944,-66.544280190716,6.));
#7219=CARTESIAN_POINT('Ctrl Pts',(0.781026555580905,-66.5463380912692,6.));
#7220=CARTESIAN_POINT('Ctrl Pts',(0.844159742305148,-66.5504744050144,6.));
#7221=CARTESIAN_POINT('Ctrl Pts',(0.907238909031849,-66.5551138190841,5.99999999999562));
#7222=CARTESIAN_POINT('Ctrl Pts',(0.970229312666943,-66.5602532333437,6.00000000002393));
#7223=CARTESIAN_POINT('Ctrl Pts',(1.16909638809118,-66.5764788839859,6.00000000011334));
#7224=CARTESIAN_POINT('Ctrl Pts',(1.36707745106602,-66.5976891098057,6.00000000097192));
#7225=CARTESIAN_POINT('Ctrl Pts',(1.56441901194577,-66.6238225866039,6.0000000005982));
#7226=CARTESIAN_POINT('Ctrl Pts',(1.69159274010741,-66.6406639030476,6.00000000035737));
#7227=CARTESIAN_POINT('Ctrl Pts',(1.81840056742283,-66.6595543873186,6.00000000016109));
#7228=CARTESIAN_POINT('Ctrl Pts',(1.94502307448575,-66.680510813247,6.00000000007684));
#7229=CARTESIAN_POINT('Ctrl Pts',(2.07712304386896,-66.7023737765363,5.99999999998895));
#7230=CARTESIAN_POINT('Ctrl Pts',(2.20902137412523,-66.7264851999825,6.));
#7231=CARTESIAN_POINT('Ctrl Pts',(2.34063577451671,-66.7528468972374,6.));
#7232=CARTESIAN_POINT('Ctrl Pts',(2.51087892012245,-66.7869457363525,6.));
#7233=CARTESIAN_POINT('Ctrl Pts',(2.68076920433902,-66.8248475460883,6.0000000000736));
#7234=CARTESIAN_POINT('Ctrl Pts',(2.84959845041541,-66.8664159843698,6.00000000019824));
#7235=CARTESIAN_POINT('Ctrl Pts',(2.86928581831134,-66.8712633266184,6.00000000021277));
#7236=CARTESIAN_POINT('Ctrl Pts',(2.88895877345423,-66.8761604719933,6.0000000002261));
#7237=CARTESIAN_POINT('Ctrl Pts',(2.9086162068755,-66.8811071600656,6.00000000023689));
#7238=CARTESIAN_POINT('Ctrl Pts',(2.97562818114549,-66.8979703652826,6.00000000027368));
#7239=CARTESIAN_POINT('Ctrl Pts',(3.0424597316486,-66.9154094072014,6.00000000027452));
#7240=CARTESIAN_POINT('Ctrl Pts',(3.1090773696706,-66.9334077173886,6.0000000002174));
#7241=CARTESIAN_POINT('Ctrl Pts',(3.33115392136444,-66.9934068824954,6.00000000002699));
#7242=CARTESIAN_POINT('Ctrl Pts',(3.55100718513146,-67.0597320616738,6.00000000008105));
#7243=CARTESIAN_POINT('Ctrl Pts',(3.76826014113968,-67.1320917176049,6.00000000079042));
#7244=CARTESIAN_POINT('Ctrl Pts',(3.79535456432316,-67.1411159590939,6.00000000087888));
#7245=CARTESIAN_POINT('Ctrl Pts',(3.82240852080627,-67.150234120291,6.00000000097954));
#7246=CARTESIAN_POINT('Ctrl Pts',(3.84942125786838,-67.1594456880511,6.00000000109367));
#7247=CARTESIAN_POINT('Ctrl Pts',(4.06549218187766,-67.2331276682562,6.00000000200657));
#7248=CARTESIAN_POINT('Ctrl Pts',(4.27892719470564,-67.3127819172318,6.00000000402309));
#7249=CARTESIAN_POINT('Ctrl Pts',(4.49003997396306,-67.3985522392496,6.00000000629976));
#7250=CARTESIAN_POINT('Ctrl Pts',(4.52450930322692,-67.4125563439803,6.00000000667148));
#7251=CARTESIAN_POINT('Ctrl Pts',(4.55891668939615,-67.4267236013019,6.00000000704364));
#7252=CARTESIAN_POINT('Ctrl Pts',(4.59326345679802,-67.4410547629658,6.0000000074056));
#7253=CARTESIAN_POINT('Ctrl Pts',(4.91663840853981,-67.5759827070503,6.00000001081344));
#7254=CARTESIAN_POINT('Ctrl Pts',(5.23400689054315,-67.7250589551412,6.00000000260231));
#7255=CARTESIAN_POINT('Ctrl Pts',(5.54574356918105,-67.888655616953,6.00000000079463));
#7256=CARTESIAN_POINT('Ctrl Pts',(5.57540428853847,-67.9042213010907,6.00000000062264));
#7257=CARTESIAN_POINT('Ctrl Pts',(5.60501398554727,-67.9199184303487,6.00000000048578));
#7258=CARTESIAN_POINT('Ctrl Pts',(5.63457295923163,-67.935747320328,6.00000000037912));
#7259=CARTESIAN_POINT('Ctrl Pts',(5.75729333486438,-68.0014643288026,5.9999999999363));
#7260=CARTESIAN_POINT('Ctrl Pts',(5.87913955282878,-68.0694525055383,6.));
#7261=CARTESIAN_POINT('Ctrl Pts',(5.9999885243854,-68.1396985954798,6.));
#7262=CARTESIAN_POINT('',(6.,-16.9705627484771,6.));
#7263=CARTESIAN_POINT('',(6.,-68.1396788547224,6.));
#7264=CARTESIAN_POINT('',(8.,-14.8323969741913,6.));
#7265=CARTESIAN_POINT('Ctrl Pts',(6.,-16.9705627484771,6.));
#7266=CARTESIAN_POINT('Ctrl Pts',(6.,-16.7029092618308,6.));
#7267=CARTESIAN_POINT('Ctrl Pts',(6.06020384677459,-16.3874179356908,6.));
#7268=CARTESIAN_POINT('Ctrl Pts',(6.25585405294364,-15.8960743911704,6.));
#7269=CARTESIAN_POINT('Ctrl Pts',(6.42385919064368,-15.6314481148128,6.));
#7270=CARTESIAN_POINT('Ctrl Pts',(6.7778910457933,-15.2614647616422,6.));
#7271=CARTESIAN_POINT('Ctrl Pts',(7.02372732242562,-15.0877073947429,6.));
#7272=CARTESIAN_POINT('Ctrl Pts',(7.47536381734142,-14.8921163084765,6.));
#7273=CARTESIAN_POINT('Ctrl Pts',(7.75869936772315,-14.8323969741913,6.));
#7274=CARTESIAN_POINT('Ctrl Pts',(8.,-14.8323969741913,6.));
#7275=CARTESIAN_POINT('',(-8.,-14.8323969741913,6.));
#7276=CARTESIAN_POINT('',(8.,-14.8323969741913,6.));
#7277=CARTESIAN_POINT('Ctrl Pts',(-8.,-14.8323969741913,6.));
#7278=CARTESIAN_POINT('Ctrl Pts',(-7.75869936772315,-14.8323969741913,6.));
#7279=CARTESIAN_POINT('Ctrl Pts',(-7.47536381734142,-14.8921163084765,6.));
#7280=CARTESIAN_POINT('Ctrl Pts',(-7.02372732242562,-15.0877073947429,6.));
#7281=CARTESIAN_POINT('Ctrl Pts',(-6.7778910457933,-15.2614647616422,6.));
#7282=CARTESIAN_POINT('Ctrl Pts',(-6.42385919064368,-15.6314481148128,6.));
#7283=CARTESIAN_POINT('Ctrl Pts',(-6.25585405294364,-15.8960743911704,6.));
#7284=CARTESIAN_POINT('Ctrl Pts',(-6.06020384677459,-16.3874179356908,6.));
#7285=CARTESIAN_POINT('Ctrl Pts',(-6.,-16.7029092618308,6.));
#7286=CARTESIAN_POINT('Ctrl Pts',(-6.,-16.9705627484771,6.));
#7287=CARTESIAN_POINT('Origin',(0.,0.,-6.));
#7288=CARTESIAN_POINT('',(6.,-68.1396788547224,-6.));
#7289=CARTESIAN_POINT('',(6.,-16.9705627484771,-6.));
#7290=CARTESIAN_POINT('',(6.,-68.1396788547224,-6.));
#7291=CARTESIAN_POINT('',(-5.99998487131667,-68.1397397005649,-6.));
#7292=CARTESIAN_POINT('Ctrl Pts',(6.,-68.1396788547224,-6.00000000013144));
#7293=CARTESIAN_POINT('Ctrl Pts',(5.88431855295697,-68.0724390389171,-6.00000000006489));
#7294=CARTESIAN_POINT('Ctrl Pts',(5.7676591844522,-68.0072232568843,-6.00000000003826));
#7295=CARTESIAN_POINT('Ctrl Pts',(5.65004937877417,-67.9440161339786,-6.00000000002279));
#7296=CARTESIAN_POINT('Ctrl Pts',(5.3937853188605,-67.8062919549623,-5.9999999999891));
#7297=CARTESIAN_POINT('Ctrl Pts',(5.13300599736668,-67.678106939822,-6.00000000000005));
#7298=CARTESIAN_POINT('Ctrl Pts',(4.86746106690753,-67.5594828278984,-6.00000000000001));
#7299=CARTESIAN_POINT('Ctrl Pts',(4.83528148125953,-67.5451075778683,-6.));
#7300=CARTESIAN_POINT('Ctrl Pts',(4.80303195584665,-67.5308726891517,-6.));
#7301=CARTESIAN_POINT('Ctrl Pts',(4.77071208279603,-67.5167781638959,-6.));
#7302=CARTESIAN_POINT('Ctrl Pts',(4.70926493087086,-67.4899813867754,-6.));
#7303=CARTESIAN_POINT('Ctrl Pts',(4.64756353476018,-67.4636919913991,-6.));
#7304=CARTESIAN_POINT('Ctrl Pts',(4.58565379486899,-67.4379245489476,-6.));
#7305=CARTESIAN_POINT('Ctrl Pts',(4.37220621964574,-67.3490855694811,-6.));
#7306=CARTESIAN_POINT('Ctrl Pts',(4.15587960441363,-67.2662786732953,-5.99999999998255));
#7307=CARTESIAN_POINT('Ctrl Pts',(3.93822708568028,-67.19008413154,-6.00000000001744));
#7308=CARTESIAN_POINT('Ctrl Pts',(3.90982152367156,-67.1801400757894,-6.000000000022));
#7309=CARTESIAN_POINT('Ctrl Pts',(3.88139333967036,-67.1703087065859,-6.00000000002801));
#7310=CARTESIAN_POINT('Ctrl Pts',(3.8529459577009,-67.1605913714033,-6.00000000003642));
#7311=CARTESIAN_POINT('Ctrl Pts',(3.85095639975222,-67.1599117587249,-6.00000000003701));
#7312=CARTESIAN_POINT('Ctrl Pts',(3.84896674789828,-67.1592327038326,-6.00000000003761));
#7313=CARTESIAN_POINT('Ctrl Pts',(3.84697700185354,-67.1585542065258,-6.00000000003822));
#7314=CARTESIAN_POINT('Ctrl Pts',(3.59854362018346,-67.0738391843207,-6.0000000001147));
#7315=CARTESIAN_POINT('Ctrl Pts',(3.34867090555795,-66.9978150100768,-6.00000000037726));
#7316=CARTESIAN_POINT('Ctrl Pts',(3.0970148955739,-66.9301251679342,-6.0000000001887));
#7317=CARTESIAN_POINT('Ctrl Pts',(3.03668686585481,-66.9138982762787,-6.00000000014349));
#7318=CARTESIAN_POINT('Ctrl Pts',(2.97625761887668,-66.8981533988812,-6.00000000011618));
#7319=CARTESIAN_POINT('Ctrl Pts',(2.91572390730768,-66.8828865048943,-6.0000000000974));
#7320=CARTESIAN_POINT('Ctrl Pts',(2.60069430807978,-66.8034345207106,-5.99999999999966));
#7321=CARTESIAN_POINT('Ctrl Pts',(2.28283573118856,-66.7369285380892,-6.00000000005431));
#7322=CARTESIAN_POINT('Ctrl Pts',(1.96249266468246,-66.6834229474773,-6.00000000017064));
#7323=CARTESIAN_POINT('Ctrl Pts',(1.83084434322121,-66.661434267436,-6.00000000021845));
#7324=CARTESIAN_POINT('Ctrl Pts',(1.69877637473924,-66.6416411401385,-6.00000000028158));
#7325=CARTESIAN_POINT('Ctrl Pts',(1.56623212057526,-66.6240628471819,-6.00000000033809));
#7326=CARTESIAN_POINT('Ctrl Pts',(1.37616567894938,-66.5988558428255,-6.00000000041912));
#7327=CARTESIAN_POINT('Ctrl Pts',(1.18527965468047,-66.5781972427926,-6.00000000005687));
#7328=CARTESIAN_POINT('Ctrl Pts',(0.993258429335491,-66.5621547406462,-6.00000000001332));
#7329=CARTESIAN_POINT('Ctrl Pts',(0.924100321934209,-66.5563768945543,-5.99999999999763));
#7330=CARTESIAN_POINT('Ctrl Pts',(0.854794973938034,-66.5511980874682,-6.));
#7331=CARTESIAN_POINT('Ctrl Pts',(0.78537729386776,-66.54662282585,-6.));
#7332=CARTESIAN_POINT('Ctrl Pts',(0.58761689227051,-66.5335886020889,-6.));
#7333=CARTESIAN_POINT('Ctrl Pts',(0.388725531373241,-66.5254312595703,-6.00000000003796));
#7334=CARTESIAN_POINT('Ctrl Pts',(0.189932702773266,-66.5222331826198,-6.00000000006191));
#7335=CARTESIAN_POINT('Ctrl Pts',(0.129733694324287,-66.5212647318828,-6.00000000006917));
#7336=CARTESIAN_POINT('Ctrl Pts',(0.0695437634146782,-66.5207506940299,
-6.00000000006915));
#7337=CARTESIAN_POINT('Ctrl Pts',(0.00939704873694772,-66.5206924120396,
-6.00000000005797));
#7338=CARTESIAN_POINT('Ctrl Pts',(0.00486457424914242,-66.5206880200851,
-6.00000000005713));
#7339=CARTESIAN_POINT('Ctrl Pts',(0.000332345131820627,-66.5206862160106,
-6.00000000005623));
#7340=CARTESIAN_POINT('Ctrl Pts',(-0.00419963646448403,-66.5206869989526,
-6.00000000005528));
#7341=CARTESIAN_POINT('Ctrl Pts',(-0.226524783799693,-66.5207254076917,
-6.0000000000086));
#7342=CARTESIAN_POINT('Ctrl Pts',(-0.448114520868727,-66.527009152027,-6.00000000000579));
#7343=CARTESIAN_POINT('Ctrl Pts',(-0.669311485207584,-66.5394717362943,
-6.00000000000955));
#7344=CARTESIAN_POINT('Ctrl Pts',(-0.770539573358165,-66.5451750857167,
-6.00000000001128));
#7345=CARTESIAN_POINT('Ctrl Pts',(-0.871685333114638,-66.5521732055682,
-6.00000000001531));
#7346=CARTESIAN_POINT('Ctrl Pts',(-0.972781317612711,-66.5604633413958,
-6.00000000003085));
#7347=CARTESIAN_POINT('Ctrl Pts',(-1.17396285232126,-66.5769607547899,-6.00000000006176));
#7348=CARTESIAN_POINT('Ctrl Pts',(-1.37494768217033,-66.598572495594,-6.00000000011194));
#7349=CARTESIAN_POINT('Ctrl Pts',(-1.57561914509455,-66.6253535036886,-6.00000000048414));
#7350=CARTESIAN_POINT('Ctrl Pts',(-1.70028466153739,-66.6419909874459,-6.00000000071536));
#7351=CARTESIAN_POINT('Ctrl Pts',(-1.82485065445227,-66.660607736393,-6.00000000050103));
#7352=CARTESIAN_POINT('Ctrl Pts',(-1.94909396401198,-66.6812022207803,-6.00000000029781));
#7353=CARTESIAN_POINT('Ctrl Pts',(-2.0848966314161,-66.7037127762663,-6.00000000007568));
#7354=CARTESIAN_POINT('Ctrl Pts',(-2.22031339976462,-66.7285864979411,-6.00000000000453));
#7355=CARTESIAN_POINT('Ctrl Pts',(-2.3549030504907,-66.7557199666411,-6.00000000000221));
#7356=CARTESIAN_POINT('Ctrl Pts',(-2.51865982162473,-66.7887335690987,-5.9999999999994));
#7357=CARTESIAN_POINT('Ctrl Pts',(-2.68130102306261,-66.8250856467162,-5.99999999999308));
#7358=CARTESIAN_POINT('Ctrl Pts',(-2.8426997479817,-66.8647055953633,-6.00000000001334));
#7359=CARTESIAN_POINT('Ctrl Pts',(-2.86572548783398,-66.8703579239735,-6.00000000001623));
#7360=CARTESIAN_POINT('Ctrl Pts',(-2.88872591532923,-66.8760768464516,-6.00000000001994));
#7361=CARTESIAN_POINT('Ctrl Pts',(-2.91170063361983,-66.8818622395366,-6.00000000002491));
#7362=CARTESIAN_POINT('Ctrl Pts',(-2.98113403408278,-66.8993466547894,-6.00000000003995));
#7363=CARTESIAN_POINT('Ctrl Pts',(-3.05033266760026,-66.9174380547095,-6.00000000006545));
#7364=CARTESIAN_POINT('Ctrl Pts',(-3.11932927971148,-66.9361435770914,-6.00000000012216));
#7365=CARTESIAN_POINT('Ctrl Pts',(-3.36477153969483,-67.0026848977026,-6.00000000032391));
#7366=CARTESIAN_POINT('Ctrl Pts',(-3.60725660149244,-67.076855084671,-6.00000000029447));
#7367=CARTESIAN_POINT('Ctrl Pts',(-3.84706864433633,-67.1586014083108,-6.00000000017254));
#7368=CARTESIAN_POINT('Ctrl Pts',(-4.09941161515419,-67.2446192325872,-6.00000000004424));
#7369=CARTESIAN_POINT('Ctrl Pts',(-4.34879490495171,-67.339026044747,-5.99999999999992));
#7370=CARTESIAN_POINT('Ctrl Pts',(-4.59498688622864,-67.4417848987278,-6.00000000000334));
#7371=CARTESIAN_POINT('Ctrl Pts',(-4.648604639256,-67.4641645831738,-6.00000000000409));
#7372=CARTESIAN_POINT('Ctrl Pts',(-4.70206437699528,-67.486936418879,-6.00000000000469));
#7373=CARTESIAN_POINT('Ctrl Pts',(-4.7553715616119,-67.510102683164,-6.00000000000505));
#7374=CARTESIAN_POINT('Ctrl Pts',(-4.93643836022568,-67.5887907875931,-6.00000000000627));
#7375=CARTESIAN_POINT('Ctrl Pts',(-5.11574645123503,-67.6720258946313,-6.00000000000435));
#7376=CARTESIAN_POINT('Ctrl Pts',(-5.29342576273543,-67.7599657462627,-6.00000000000267));
#7377=CARTESIAN_POINT('Ctrl Pts',(-5.40844988249057,-67.8168953006373,-6.00000000000159));
#7378=CARTESIAN_POINT('Ctrl Pts',(-5.52279105849346,-67.8757975188366,-6.00000000000073));
#7379=CARTESIAN_POINT('Ctrl Pts',(-5.63648028596659,-67.9367260770655,-6.00000000000035));
#7380=CARTESIAN_POINT('Ctrl Pts',(-5.75848075352519,-68.0021088117081,-5.99999999999995));
#7381=CARTESIAN_POINT('Ctrl Pts',(-5.87973098327784,-68.0698251706507,-6.));
#7382=CARTESIAN_POINT('Ctrl Pts',(-5.99996974263335,-68.1397309048551,-6.));
#7383=CARTESIAN_POINT('',(-5.99999999999999,-16.9705627484771,-6.));
#7384=CARTESIAN_POINT('',(-5.99999999999999,-16.9705627484771,-6.));
#7385=CARTESIAN_POINT('',(-7.99999999999999,-14.8323969741913,-6.));
#7386=CARTESIAN_POINT('Ctrl Pts',(-6.,-16.9705627484771,-6.));
#7387=CARTESIAN_POINT('Ctrl Pts',(-6.,-16.7029092618308,-6.));
#7388=CARTESIAN_POINT('Ctrl Pts',(-6.06020384677459,-16.3874179356908,-6.));
#7389=CARTESIAN_POINT('Ctrl Pts',(-6.25585405294364,-15.8960743911704,-6.));
#7390=CARTESIAN_POINT('Ctrl Pts',(-6.42385919064368,-15.6314481148128,-6.));
#7391=CARTESIAN_POINT('Ctrl Pts',(-6.7778910457933,-15.2614647616422,-6.));
#7392=CARTESIAN_POINT('Ctrl Pts',(-7.02372732242562,-15.0877073947429,-6.));
#7393=CARTESIAN_POINT('Ctrl Pts',(-7.47536381734142,-14.8921163084765,-6.));
#7394=CARTESIAN_POINT('Ctrl Pts',(-7.75869936772315,-14.8323969741913,-6.));
#7395=CARTESIAN_POINT('Ctrl Pts',(-8.,-14.8323969741913,-6.));
#7396=CARTESIAN_POINT('',(8.,-14.8323969741913,-6.));
#7397=CARTESIAN_POINT('',(8.,-14.8323969741913,-6.));
#7398=CARTESIAN_POINT('Ctrl Pts',(8.,-14.8323969741913,-6.));
#7399=CARTESIAN_POINT('Ctrl Pts',(7.75869936772315,-14.8323969741913,-6.));
#7400=CARTESIAN_POINT('Ctrl Pts',(7.47536381734142,-14.8921163084765,-6.));
#7401=CARTESIAN_POINT('Ctrl Pts',(7.02372732242562,-15.0877073947429,-6.));
#7402=CARTESIAN_POINT('Ctrl Pts',(6.7778910457933,-15.2614647616422,-6.));
#7403=CARTESIAN_POINT('Ctrl Pts',(6.42385919064368,-15.6314481148128,-6.));
#7404=CARTESIAN_POINT('Ctrl Pts',(6.25585405294364,-15.8960743911704,-6.));
#7405=CARTESIAN_POINT('Ctrl Pts',(6.06020384677459,-16.3874179356908,-6.));
#7406=CARTESIAN_POINT('Ctrl Pts',(6.,-16.7029092618308,-6.));
#7407=CARTESIAN_POINT('Ctrl Pts',(6.,-16.9705627484771,-6.));
#7408=CARTESIAN_POINT('Origin',(6.,-81.,6.));
#7409=CARTESIAN_POINT('Origin',(6.,0.,0.));
#7410=CARTESIAN_POINT('',(5.99999997747517,-70.5266986161245,8.18443785141233));
#7411=CARTESIAN_POINT('Ctrl Pts',(6.,-68.1397047377494,6.00000000000005));
#7412=CARTESIAN_POINT('Ctrl Pts',(6.,-68.4373158828193,5.99999994125204));
#7413=CARTESIAN_POINT('Ctrl Pts',(6.,-68.7350865689403,6.04968588989578));
#7414=CARTESIAN_POINT('Ctrl Pts',(6.,-69.3065983612443,6.24469586989208));
#7415=CARTESIAN_POINT('Ctrl Pts',(6.00000000000086,-69.5806827235788,6.39330918939534));
#7416=CARTESIAN_POINT('Ctrl Pts',(6.00000000000086,-70.0282142371682,6.76203382605757));
#7417=CARTESIAN_POINT('Ctrl Pts',(6.,-70.2089115578842,6.97327876337078));
#7418=CARTESIAN_POINT('Ctrl Pts',(6.,-70.419255711698,7.36995744983913));
#7419=CARTESIAN_POINT('Ctrl Pts',(6.00000000004193,-70.478593909457,7.53530402271511));
#7420=CARTESIAN_POINT('Ctrl Pts',(6.00000000004193,-70.5396316268949,7.86534218943114));
#7421=CARTESIAN_POINT('Ctrl Pts',(6.,-70.5451733494511,8.02524609190228));
#7422=CARTESIAN_POINT('Ctrl Pts',(6.,-70.5267003657195,8.1844379608027));
#7423=CARTESIAN_POINT('',(6.,-70.5266968882288,-8.18443804032376));
#7424=CARTESIAN_POINT('Origin',(6.,0.,0.));
#7425=CARTESIAN_POINT('Ctrl Pts',(6.,-70.5266941883794,-8.1844377270085));
#7426=CARTESIAN_POINT('Ctrl Pts',(6.,-70.545094155265,-8.02588689619588));
#7427=CARTESIAN_POINT('Ctrl Pts',(6.00000000000071,-70.5396715184363,-7.8666208745049));
#7428=CARTESIAN_POINT('Ctrl Pts',(6.00000000000071,-70.4792696976785,-7.53789411375645));
#7429=CARTESIAN_POINT('Ctrl Pts',(5.99999999997532,-70.4204873797258,-7.3731678146394));
#7430=CARTESIAN_POINT('Ctrl Pts',(5.99999999997532,-70.2115377007883,-6.97699421954287));
#7431=CARTESIAN_POINT('Ctrl Pts',(6.0000000000039,-70.0315342165176,-6.76562661457263));
#7432=CARTESIAN_POINT('Ctrl Pts',(6.0000000000039,-69.5852755560958,-6.3962832399853));
#7433=CARTESIAN_POINT('Ctrl Pts',(6.,-69.3117412488074,-6.24719387088984));
#7434=CARTESIAN_POINT('Ctrl Pts',(6.,-68.7390122653034,-6.05035683158401));
#7435=CARTESIAN_POINT('Ctrl Pts',(6.,-68.4392574758577,-6.00000296963229));
#7436=CARTESIAN_POINT('Ctrl Pts',(6.,-68.1396788547224,-6.00000000013144));
#7437=CARTESIAN_POINT('Origin',(6.,-81.,6.));
#7438=CARTESIAN_POINT('',(6.,5.99999999999994,-16.9705627484772));
#7439=CARTESIAN_POINT('',(6.00000000000004,6.00000000137574,-68.1396788547223));
#7440=CARTESIAN_POINT('',(6.,5.99999999999994,-16.9705627484772));
#7441=CARTESIAN_POINT('',(6.,-6.00000000000006,-16.9705627484771));
#7442=CARTESIAN_POINT('Origin',(6.,0.,0.));
#7443=CARTESIAN_POINT('',(6.,-6.00000000000024,-68.1396788547224));
#7444=CARTESIAN_POINT('',(6.,-6.00000000000006,-16.9705627484771));
#7445=CARTESIAN_POINT('',(5.99999998184743,-8.18443790004951,-70.5266981504358));
#7446=CARTESIAN_POINT('Ctrl Pts',(6.,-6.00000000014129,-68.1396788547224));
#7447=CARTESIAN_POINT('Ctrl Pts',(6.,-6.00000305608312,-68.4373010930767));
#7448=CARTESIAN_POINT('Ctrl Pts',(6.,-6.04969479661867,-68.7350934660561));
#7449=CARTESIAN_POINT('Ctrl Pts',(6.,-6.24470400429899,-69.3066252131869));
#7450=CARTESIAN_POINT('Ctrl Pts',(6.00000000000098,-6.3933099872563,-69.5806863242555));
#7451=CARTESIAN_POINT('Ctrl Pts',(6.00000000000098,-6.76203851696321,-70.0282149179196));
#7452=CARTESIAN_POINT('Ctrl Pts',(6.,-6.97329170868472,-70.2089173284816));
#7453=CARTESIAN_POINT('Ctrl Pts',(6.,-7.36997476707013,-70.4192602993792));
#7454=CARTESIAN_POINT('Ctrl Pts',(6.00000000002305,-7.5353194148801,-70.4785967892622));
#7455=CARTESIAN_POINT('Ctrl Pts',(6.00000000002305,-7.86535152657698,-70.539631175309));
#7456=CARTESIAN_POINT('Ctrl Pts',(6.,-8.02525083439126,-70.5451720759936));
#7457=CARTESIAN_POINT('Ctrl Pts',(6.,-8.18443797997434,-70.5266994310349));
#7458=CARTESIAN_POINT('',(6.,-8.69499227394621E-15,-71.));
#7459=CARTESIAN_POINT('Origin',(6.,0.,0.));
#7460=CARTESIAN_POINT('',(6.,8.18443804021865,-70.526696888241));
#7461=CARTESIAN_POINT('Origin',(6.,0.,0.));
#7462=CARTESIAN_POINT('Ctrl Pts',(6.,8.18443732241168,-70.5266907030083));
#7463=CARTESIAN_POINT('Ctrl Pts',(6.,8.02588523103638,-70.5450916207373));
#7464=CARTESIAN_POINT('Ctrl Pts',(5.99999999999586,7.86661749518644,-70.5396685015587));
#7465=CARTESIAN_POINT('Ctrl Pts',(5.99999999999586,7.53788974855862,-70.4792626150954));
#7466=CARTESIAN_POINT('Ctrl Pts',(6.00000000013518,7.37316514653039,-70.4204769991494));
#7467=CARTESIAN_POINT('Ctrl Pts',(6.00000000013518,6.97700277618102,-70.2115159486837));
#7468=CARTESIAN_POINT('Ctrl Pts',(6.00000000002034,6.76564989236828,-70.031506529363));
#7469=CARTESIAN_POINT('Ctrl Pts',(6.00000000002034,6.39630460490681,-69.5852188894777));
#7470=CARTESIAN_POINT('Ctrl Pts',(6.,6.2472019641686,-69.3116452689945));
#7471=CARTESIAN_POINT('Ctrl Pts',(6.,6.0503726902255,-68.7389238969686));
#7472=CARTESIAN_POINT('Ctrl Pts',(6.,6.0000144140978,-68.4392189678418));
#7473=CARTESIAN_POINT('Ctrl Pts',(6.,6.00000000309571,-68.1396788547223));
#7474=CARTESIAN_POINT('Origin',(6.,-81.,6.));
#7475=CARTESIAN_POINT('',(6.,16.9705627484771,6.));
#7476=CARTESIAN_POINT('',(6.,68.1396788547224,6.));
#7477=CARTESIAN_POINT('',(6.,16.9705627484771,6.));
#7478=CARTESIAN_POINT('',(6.,16.9705627484771,-6.));
#7479=CARTESIAN_POINT('Origin',(6.,0.,0.));
#7480=CARTESIAN_POINT('',(6.,68.1396788547224,-6.));
#7481=CARTESIAN_POINT('',(6.,16.9705627484771,-6.));
#7482=CARTESIAN_POINT('',(5.99999996627066,70.5266997009286,-8.18443773117988));
#7483=CARTESIAN_POINT('Ctrl Pts',(6.,68.1396788547224,-6.00000000027673));
#7484=CARTESIAN_POINT('Ctrl Pts',(6.,68.4373270704393,-6.00000428105949));
#7485=CARTESIAN_POINT('Ctrl Pts',(6.,68.7351416846738,-6.04970657903531));
#7486=CARTESIAN_POINT('Ctrl Pts',(6.,69.3066578408989,-6.24472384735339));
#7487=CARTESIAN_POINT('Ctrl Pts',(6.00000000000379,69.5807112996191,-6.39331409080519));
#7488=CARTESIAN_POINT('Ctrl Pts',(6.00000000000379,70.0282207454831,-6.76201643771438));
#7489=CARTESIAN_POINT('Ctrl Pts',(6.,70.2089084902967,-6.97325603566953));
#7490=CARTESIAN_POINT('Ctrl Pts',(6.,70.4192518011347,-7.36993244016015));
#7491=CARTESIAN_POINT('Ctrl Pts',(6.00000000005203,70.4785926358654,-7.53528540527057));
#7492=CARTESIAN_POINT('Ctrl Pts',(6.00000000005203,70.5396331215713,-7.86533365840252));
#7493=CARTESIAN_POINT('Ctrl Pts',(6.,70.5451755297387,-8.02524154134083));
#7494=CARTESIAN_POINT('Ctrl Pts',(6.,70.5267025420345,-8.18443790911504));
#7495=CARTESIAN_POINT('',(6.,70.5266968882319,8.1844380402973));
#7496=CARTESIAN_POINT('Origin',(6.,0.,0.));
#7497=CARTESIAN_POINT('Ctrl Pts',(6.,70.5266929827526,8.18443758706622));
#7498=CARTESIAN_POINT('Ctrl Pts',(6.,70.5450932974979,8.0258861584249));
#7499=CARTESIAN_POINT('Ctrl Pts',(5.99999999999889,70.5396704643105,7.86661938607951));
#7500=CARTESIAN_POINT('Ctrl Pts',(5.99999999999889,70.4792671686154,7.53789242311621));
#7501=CARTESIAN_POINT('Ctrl Pts',(6.00000000003674,70.4204838116755,7.37316698642186));
#7502=CARTESIAN_POINT('Ctrl Pts',(6.00000000003674,70.2115304106972,6.97699734385621));
#7503=CARTESIAN_POINT('Ctrl Pts',(6.00000000000814,70.0315248324418,6.76563460399418));
#7504=CARTESIAN_POINT('Ctrl Pts',(6.00000000000814,69.5852562206707,6.39629025610278));
#7505=CARTESIAN_POINT('Ctrl Pts',(6.,69.3117083967071,6.24719613036894));
#7506=CARTESIAN_POINT('Ctrl Pts',(6.,68.7389797637441,6.05036104748683));
#7507=CARTESIAN_POINT('Ctrl Pts',(6.,68.4392465048021,6.00000664112192));
#7508=CARTESIAN_POINT('Ctrl Pts',(6.,68.1396788547224,6.00000000065731));
#7509=CARTESIAN_POINT('Origin',(-6.,81.,6.));
#7510=CARTESIAN_POINT('',(-5.99999290989181,-6.00000000000024,-68.1397216273217));
#7511=CARTESIAN_POINT('',(-6.,-6.00000000000006,-16.9705627484771));
#7512=CARTESIAN_POINT('',(-6.,-6.00000000000024,-68.1396788547224));
#7513=CARTESIAN_POINT('',(-6.,5.99999999999994,-16.9705627484772));
#7514=CARTESIAN_POINT('Origin',(-6.,1.17789865652746E-16,0.));
#7515=CARTESIAN_POINT('',(-6.00000000000002,6.00000000097442,-68.1396788547224));
#7516=CARTESIAN_POINT('',(-6.,5.99999999999976,-68.1396788547224));
#7517=CARTESIAN_POINT('',(-6.00000002824202,8.1844377839641,-70.5266946795513));
#7518=CARTESIAN_POINT('Ctrl Pts',(-6.,6.00000000292373,-68.1396788547223));
#7519=CARTESIAN_POINT('Ctrl Pts',(-6.,6.00001391381448,-68.4372133964188));
#7520=CARTESIAN_POINT('Ctrl Pts',(-5.99999999999999,6.04969606840112,-68.7349087606943));
#7521=CARTESIAN_POINT('Ctrl Pts',(-5.99999999999999,6.24468515704947,-69.3064384243037));
#7522=CARTESIAN_POINT('Ctrl Pts',(-6.0000000000128,6.39333208418984,-69.5805779022244));
#7523=CARTESIAN_POINT('Ctrl Pts',(-6.0000000000128,6.76209102052247,-70.0281703224301));
#7524=CARTESIAN_POINT('Ctrl Pts',(-6.00000000005601,6.97333367723825,-70.2088938300498));
#7525=CARTESIAN_POINT('Ctrl Pts',(-6.00000000005601,7.37000454340887,-70.4192521725936));
#7526=CARTESIAN_POINT('Ctrl Pts',(-5.999999999998,7.53533754904914,-70.4785892063122));
#7527=CARTESIAN_POINT('Ctrl Pts',(-5.999999999998,7.86535726226597,-70.539625540259));
#7528=CARTESIAN_POINT('Ctrl Pts',(-6.,8.025254109816,-70.5451662722122));
#7529=CARTESIAN_POINT('Ctrl Pts',(-6.,8.18443751976133,-70.5266924030008));
#7530=CARTESIAN_POINT('',(-6.,-8.69499227394621E-15,-71.));
#7531=CARTESIAN_POINT('Origin',(-6.,1.23378335349421E-30,3.53369596958238E-16));
#7532=CARTESIAN_POINT('',(-6.,-8.18443766083924,-70.526696932267));
#7533=CARTESIAN_POINT('Origin',(-6.,1.23378335349421E-30,3.53369596958238E-16));
#7534=CARTESIAN_POINT('Ctrl Pts',(-5.99999999999999,-8.18443796501575,-70.526700334414));
#7535=CARTESIAN_POINT('Ctrl Pts',(-5.99999999999999,-8.02587645834891,-70.5451002268863));
#7536=CARTESIAN_POINT('Ctrl Pts',(-6.00000000003802,-7.86660059219007,-70.5396760412271));
#7537=CARTESIAN_POINT('Ctrl Pts',(-6.00000000003802,-7.53785319168903,-70.4792688770294));
#7538=CARTESIAN_POINT('Ctrl Pts',(-5.99999999999999,-7.37311459450185,-70.4204826109743));
#7539=CARTESIAN_POINT('Ctrl Pts',(-5.99999999999999,-6.97694305312581,-70.2115379778568));
#7540=CARTESIAN_POINT('Ctrl Pts',(-6.00000000000057,-6.76558623416905,-70.0315567355748));
#7541=CARTESIAN_POINT('Ctrl Pts',(-6.00000000000057,-6.39627508448911,-69.5853337607453));
#7542=CARTESIAN_POINT('Ctrl Pts',(-5.99999999999999,-6.24720735674295,-69.3118178138716));
#7543=CARTESIAN_POINT('Ctrl Pts',(-5.99999999999999,-6.05035981119347,-68.7391217993171));
#7544=CARTESIAN_POINT('Ctrl Pts',(-5.99999999999999,-6.00000000000023,-68.4393438744497));
#7545=CARTESIAN_POINT('Ctrl Pts',(-5.99999999999999,-6.00000000000024,-68.1397278083536));
#7546=CARTESIAN_POINT('Origin',(-6.,81.,6.));
#7547=CARTESIAN_POINT('Origin',(-6.,1.17789865652746E-16,0.));
#7548=CARTESIAN_POINT('',(-6.00000002044165,-70.5266952569886,-8.18443785100741));
#7549=CARTESIAN_POINT('Ctrl Pts',(-5.99999999999999,-68.1397484962748,-6.));
#7550=CARTESIAN_POINT('Ctrl Pts',(-5.99999999999999,-68.4372667215367,-6.));
#7551=CARTESIAN_POINT('Ctrl Pts',(-5.99999999999999,-68.7349424975465,-6.04964870253574));
#7552=CARTESIAN_POINT('Ctrl Pts',(-5.99999999999999,-69.3064745088027,-6.24462699368351));
#7553=CARTESIAN_POINT('Ctrl Pts',(-6.00000000000153,-69.5806092392168,-6.39328901413462));
#7554=CARTESIAN_POINT('Ctrl Pts',(-6.00000000000153,-70.0282000466676,-6.76208375846719));
#7555=CARTESIAN_POINT('Ctrl Pts',(-6.00000000035957,-70.2089294430131,-6.9733562678496));
#7556=CARTESIAN_POINT('Ctrl Pts',(-6.00000000035957,-70.4192721255049,-7.37004589750889));
#7557=CARTESIAN_POINT('Ctrl Pts',(-5.99999999998651,-70.4786003297255,-7.53537093001657));
#7558=CARTESIAN_POINT('Ctrl Pts',(-5.99999999998651,-70.5396271011112,-7.8653738247129));
#7559=CARTESIAN_POINT('Ctrl Pts',(-5.99999999999999,-70.5451662208239,-8.0252622570676));
#7560=CARTESIAN_POINT('Ctrl Pts',(-5.99999999999999,-70.5266935751337,-8.18443765582455));
#7561=CARTESIAN_POINT('',(-5.99999998001766,-70.5266982778411,8.18443788597873));
#7562=CARTESIAN_POINT('Origin',(-6.,-3.53369596958238E-16,0.));
#7563=CARTESIAN_POINT('Ctrl Pts',(-5.99999999999999,-70.5266996874987,8.18443797574402));
#7564=CARTESIAN_POINT('Ctrl Pts',(-5.99999999999999,-70.5450992579752,8.0258803335721));
#7565=CARTESIAN_POINT('Ctrl Pts',(-6.00000000002134,-70.5396757507429,7.86660830835082));
#7566=CARTESIAN_POINT('Ctrl Pts',(-6.00000000002134,-70.4792714259724,7.53786559283121));
#7567=CARTESIAN_POINT('Ctrl Pts',(-5.99999999999999,-70.42048657203,7.37312821110373));
#7568=CARTESIAN_POINT('Ctrl Pts',(-5.99999999999999,-70.2115435781299,6.97695270225775));
#7569=CARTESIAN_POINT('Ctrl Pts',(-6.00000000000098,-70.031558716588,6.76558800338714));
#7570=CARTESIAN_POINT('Ctrl Pts',(-6.00000000000098,-69.5853412925519,6.39627546000802));
#7571=CARTESIAN_POINT('Ctrl Pts',(-5.99999999999999,-69.3118535798659,6.24721921781684));
#7572=CARTESIAN_POINT('Ctrl Pts',(-5.99999999999999,-68.739127923668,6.05037041272747));
#7573=CARTESIAN_POINT('Ctrl Pts',(-5.99999999999999,-68.4393146647117,6.00000293652382));
#7574=CARTESIAN_POINT('Ctrl Pts',(-5.99999999999999,-68.1396788547224,6.00000000012849));
#7575=CARTESIAN_POINT('Origin',(-6.,81.,6.));
#7576=CARTESIAN_POINT('',(-5.99999999999999,6.00000000000006,16.9705627484771));
#7577=CARTESIAN_POINT('',(-5.99999999999999,6.00000000000024,68.1396788547224));
#7578=CARTESIAN_POINT('',(-5.99999999999999,6.00000000000006,16.9705627484771));
#7579=CARTESIAN_POINT('',(-5.99999999999999,-5.99999999999994,16.9705627484772));
#7580=CARTESIAN_POINT('Origin',(-6.,1.17789865652746E-16,0.));
#7581=CARTESIAN_POINT('',(-5.99999800383455,-5.99999999999981,68.1396904583549));
#7582=CARTESIAN_POINT('',(-5.99999999999999,-5.99999999999994,16.9705627484772));
#7583=CARTESIAN_POINT('',(-5.99999997386433,-8.18443780213022,70.5266990636957));
#7584=CARTESIAN_POINT('Ctrl Pts',(-5.99999999999999,-5.99999999999991,68.1396917580846));
#7585=CARTESIAN_POINT('Ctrl Pts',(-5.99999999999999,-5.99999990221501,68.4373180189636));
#7586=CARTESIAN_POINT('Ctrl Pts',(-6.,-6.04969214680078,68.73510741349));
#7587=CARTESIAN_POINT('Ctrl Pts',(-6.,-6.24470617061769,69.3066184436945));
#7588=CARTESIAN_POINT('Ctrl Pts',(-6.00000000000163,-6.39331179161704,69.5806934109985));
#7589=CARTESIAN_POINT('Ctrl Pts',(-6.00000000000163,-6.76202707922547,70.0282163865669));
#7590=CARTESIAN_POINT('Ctrl Pts',(-5.99999999999999,-6.97326897652041,70.2089096425642));
#7591=CARTESIAN_POINT('Ctrl Pts',(-5.99999999999999,-7.36994644175672,70.4192537935309));
#7592=CARTESIAN_POINT('Ctrl Pts',(-6.00000000004821,-7.53529576254731,70.4785932103609));
#7593=CARTESIAN_POINT('Ctrl Pts',(-6.00000000004821,-7.86533835046211,70.5396322309098));
#7594=CARTESIAN_POINT('Ctrl Pts',(-6.,-8.02524406228223,70.5451742661205));
#7595=CARTESIAN_POINT('Ctrl Pts',(-6.,-8.18443793975999,70.5267012613836));
#7596=CARTESIAN_POINT('',(-6.00000002044842,8.18443786845297,70.5266954072364));
#7597=CARTESIAN_POINT('Origin',(-6.,1.23378335349421E-30,3.53369596958238E-16));
#7598=CARTESIAN_POINT('Ctrl Pts',(-6.,8.1844376908963,70.5266938772528));
#7599=CARTESIAN_POINT('Ctrl Pts',(-6.,8.02588660831281,70.545093945321));
#7600=CARTESIAN_POINT('Ctrl Pts',(-6.00000000000021,7.86662029545443,70.5396712396839));
#7601=CARTESIAN_POINT('Ctrl Pts',(-6.00000000000021,7.53789345525426,70.4792689721846));
#7602=CARTESIAN_POINT('Ctrl Pts',(-5.99999999999207,7.37316744126058,70.4204863862969));
#7603=CARTESIAN_POINT('Ctrl Pts',(-5.99999999999207,6.97699496825595,70.2115357634242));
#7604=CARTESIAN_POINT('Ctrl Pts',(-6.00000000000484,6.7656286627794,70.0315317575654));
#7605=CARTESIAN_POINT('Ctrl Pts',(-6.00000000000484,6.39628501585991,69.5852704695977));
#7606=CARTESIAN_POINT('Ctrl Pts',(-5.99999999999999,6.24719439633593,69.3117325652093));
#7607=CARTESIAN_POINT('Ctrl Pts',(-5.99999999999999,6.05035712202607,68.7390013313318));
#7608=CARTESIAN_POINT('Ctrl Pts',(-5.99999999999999,6.0000039352936,68.4392570047814));
#7609=CARTESIAN_POINT('Ctrl Pts',(-5.99999999999999,6.00000000023106,68.1396788547224));
#7610=CARTESIAN_POINT('Origin',(0.,0.,6.));
#7611=CARTESIAN_POINT('',(-5.99999659392154,68.1396991687892,6.00000000000001));
#7612=CARTESIAN_POINT('Ctrl Pts',(6.00000000000002,68.1396788547224,6.00000000065731));
#7613=CARTESIAN_POINT('Ctrl Pts',(5.88458780655166,68.0725952090573,6.0000000003255));
#7614=CARTESIAN_POINT('Ctrl Pts',(5.7681428376056,68.0075008237318,6.00000000024891));
#7615=CARTESIAN_POINT('Ctrl Pts',(5.65067183885126,67.9443722158119,6.00000000020361));
#7616=CARTESIAN_POINT('Ctrl Pts',(5.38642690984633,67.8023676811193,6.00000000010169));
#7617=CARTESIAN_POINT('Ctrl Pts',(5.11699288348237,67.6703133164605,6.00000000024462));
#7618=CARTESIAN_POINT('Ctrl Pts',(4.84313854685597,67.5486842141237,6.00000000017594));
#7619=CARTESIAN_POINT('Ctrl Pts',(4.81851114481416,67.5377462503867,6.00000000016977));
#7620=CARTESIAN_POINT('Ctrl Pts',(4.79384797350979,67.526892570235,6.00000000016207));
#7621=CARTESIAN_POINT('Ctrl Pts',(4.76914957931904,67.5161235029138,6.00000000015292));
#7622=CARTESIAN_POINT('Ctrl Pts',(4.70749169934415,67.4892392506337,6.00000000013006));
#7623=CARTESIAN_POINT('Ctrl Pts',(4.64561433330076,67.4628823302612,6.00000000009686));
#7624=CARTESIAN_POINT('Ctrl Pts',(4.58355358413935,67.4370609019436,6.00000000006413));
#7625=CARTESIAN_POINT('Ctrl Pts',(4.3984410260912,67.3600416794412,5.99999999996652));
#7626=CARTESIAN_POINT('Ctrl Pts',(4.21149574112703,67.2877208487954,5.9999999999379));
#7627=CARTESIAN_POINT('Ctrl Pts',(4.02339026402838,67.220280599234,6.00000000006967));
#7628=CARTESIAN_POINT('Ctrl Pts',(3.96640526002753,67.1998501314435,6.00000000010959));
#7629=CARTESIAN_POINT('Ctrl Pts',(3.90931362085271,67.1798679001431,6.0000000001777));
#7630=CARTESIAN_POINT('Ctrl Pts',(3.85213373160562,67.1603398560627,6.00000000033226));
#7631=CARTESIAN_POINT('Ctrl Pts',(3.85016142643025,67.1596662754924,6.0000000003376));
#7632=CARTESIAN_POINT('Ctrl Pts',(3.84818901625124,67.1589932353419,6.00000000034303));
#7633=CARTESIAN_POINT('Ctrl Pts',(3.84621650069232,67.1583207354738,6.00000000034858));
#7634=CARTESIAN_POINT('Ctrl Pts',(3.5982890765688,67.0737935644395,6.00000000104606));
#7635=CARTESIAN_POINT('Ctrl Pts',(3.3486968786768,66.9978617665185,6.00000001076173));
#7636=CARTESIAN_POINT('Ctrl Pts',(3.09725398859764,66.9301813536615,6.00000001025565));
#7637=CARTESIAN_POINT('Ctrl Pts',(2.76617148958911,66.8410644960898,6.00000000958927));
#7638=CARTESIAN_POINT('Ctrl Pts',(2.43192850502006,66.7664323064067,6.00000000286088));
#7639=CARTESIAN_POINT('Ctrl Pts',(2.09397569559093,66.706165144386,6.00000000174086));
#7640=CARTESIAN_POINT('Ctrl Pts',(2.05038959937716,66.6983924310098,6.00000000159641));
#7641=CARTESIAN_POINT('Ctrl Pts',(2.00674184718961,66.6908587070349,6.00000000150129));
#7642=CARTESIAN_POINT('Ctrl Pts',(1.96303130641295,66.6835637569233,6.00000000145524));
#7643=CARTESIAN_POINT('Ctrl Pts',(1.83087276517514,66.6615075217903,6.00000000131602));
#7644=CARTESIAN_POINT('Ctrl Pts',(1.69814016267927,66.6416339787774,6.00000000143221));
#7645=CARTESIAN_POINT('Ctrl Pts',(1.56485129042034,66.6239976603168,6.00000000294475));
#7646=CARTESIAN_POINT('Ctrl Pts',(1.37465928224473,66.5988321174775,6.00000000510302));
#7647=CARTESIAN_POINT('Ctrl Pts',(1.18358970013618,66.5781827823755,6.00000000620398));
#7648=CARTESIAN_POINT('Ctrl Pts',(0.991617758843105,66.5621619254138,6.0000000057091));
#7649=CARTESIAN_POINT('Ctrl Pts',(0.740815052328747,66.5412313964019,6.00000000506256));
#7650=CARTESIAN_POINT('Ctrl Pts',(0.488472212738995,66.5281989642491,6.00000000262167));
#7651=CARTESIAN_POINT('Ctrl Pts',(0.236328250644454,66.523133255531,6.00000000145786));
#7652=CARTESIAN_POINT('Ctrl Pts',(0.159870466408439,66.5215971772488,6.00000000110496));
#7653=CARTESIAN_POINT('Ctrl Pts',(0.0834309792026766,66.5207939914652,6.00000000083788));
#7654=CARTESIAN_POINT('Ctrl Pts',(0.00705844255551847,66.5207265533995,
6.00000000064985));
#7655=CARTESIAN_POINT('Ctrl Pts',(0.00181350859966491,66.5207219220462,
6.00000000063694));
#7656=CARTESIAN_POINT('Ctrl Pts',(-0.00343110952298811,66.5207207609042,
6.00000000062438));
#7657=CARTESIAN_POINT('Ctrl Pts',(-0.00867542023187034,66.5207230706085,
6.00000000061218));
#7658=CARTESIAN_POINT('Ctrl Pts',(-0.331628834827677,66.5208653060567,5.99999999986073));
#7659=CARTESIAN_POINT('Ctrl Pts',(-0.653114357046965,66.5341608814007,6.00000000001333));
#7660=CARTESIAN_POINT('Ctrl Pts',(-0.974743165742799,66.560621565599,6.00000000001792));
#7661=CARTESIAN_POINT('Ctrl Pts',(-1.17715728160842,66.5772743524525,6.00000000002081));
#7662=CARTESIAN_POINT('Ctrl Pts',(-1.37962806781815,66.5991418583686,6.00000000003358));
#7663=CARTESIAN_POINT('Ctrl Pts',(-1.58132881881509,66.6261417714914,6.00000000014743));
#7664=CARTESIAN_POINT('Ctrl Pts',(-1.70522987986189,66.6427273214586,6.00000000021737));
#7665=CARTESIAN_POINT('Ctrl Pts',(-1.82905078205798,66.6612792878494,6.00000000033522));
#7666=CARTESIAN_POINT('Ctrl Pts',(-1.95241072789507,66.6817574578459,6.00000000038641));
#7667=CARTESIAN_POINT('Ctrl Pts',(-2.08900850840277,66.7044331533596,6.00000000044308));
#7668=CARTESIAN_POINT('Ctrl Pts',(-2.2250405745722,66.7294710847112,6.00000000035428));
#7669=CARTESIAN_POINT('Ctrl Pts',(-2.3601828255349,66.7567627898884,6.00000000017272));
#7670=CARTESIAN_POINT('Ctrl Pts',(-2.52887378089362,66.7908295882947,5.99999999994608));
#7671=CARTESIAN_POINT('Ctrl Pts',(-2.69612953033057,66.8284193088917,6.00000000000241));
#7672=CARTESIAN_POINT('Ctrl Pts',(-2.86209194811488,66.8694715270266,6.00000000000268));
#7673=CARTESIAN_POINT('Ctrl Pts',(-2.87883967552237,66.8736142201012,6.00000000000271));
#7674=CARTESIAN_POINT('Ctrl Pts',(-2.89557422162999,66.8777922154813,6.00000000000284));
#7675=CARTESIAN_POINT('Ctrl Pts',(-2.91229572454255,66.8820054793396,6.00000000000307));
#7676=CARTESIAN_POINT('Ctrl Pts',(-2.9825032438285,66.8996954444783,6.00000000000407));
#7677=CARTESIAN_POINT('Ctrl Pts',(-3.0524808714627,66.9180070193092,6.00000000000678));
#7678=CARTESIAN_POINT('Ctrl Pts',(-3.12225265070286,66.9369440322735,6.00000000001525));
#7679=CARTESIAN_POINT('Ctrl Pts',(-3.36632242546284,67.0031878996244,6.0000000000449));
#7680=CARTESIAN_POINT('Ctrl Pts',(-3.60783909617146,67.0770801580024,6.00000000017843));
#7681=CARTESIAN_POINT('Ctrl Pts',(-3.84666540906819,67.1584730795796,6.00000000030431));
#7682=CARTESIAN_POINT('Ctrl Pts',(-4.07435177258606,67.2360694637687,6.00000000042432));
#7683=CARTESIAN_POINT('Ctrl Pts',(-4.29959331275655,67.3204828589082,6.00000000045655));
#7684=CARTESIAN_POINT('Ctrl Pts',(-4.52242840730631,67.4117842364616,6.00000000027812));
#7685=CARTESIAN_POINT('Ctrl Pts',(-4.54672655587405,67.4217398246543,6.00000000025867));
#7686=CARTESIAN_POINT('Ctrl Pts',(-4.57099610644136,67.4317772614459,6.00000000023763));
#7687=CARTESIAN_POINT('Ctrl Pts',(-4.59523711898079,67.4418966025886,6.0000000002158));
#7688=CARTESIAN_POINT('Ctrl Pts',(-4.64891007134559,67.464302222578,6.00000000016746));
#7689=CARTESIAN_POINT('Ctrl Pts',(-4.70242464530625,67.4871028602993,6.00000000013265));
#7690=CARTESIAN_POINT('Ctrl Pts',(-4.75579883589029,67.5103059640663,6.0000000001061));
#7691=CARTESIAN_POINT('Ctrl Pts',(-4.90528832196,67.5752928054479,6.00000000003174));
#7692=CARTESIAN_POINT('Ctrl Pts',(-5.05367780331171,67.6434327643659,6.0000000000171));
#7693=CARTESIAN_POINT('Ctrl Pts',(-5.20095707175058,67.7147496307297,6.00000000000847));
#7694=CARTESIAN_POINT('Ctrl Pts',(-5.34823634018945,67.7860664970935,5.99999999999985));
#7695=CARTESIAN_POINT('Ctrl Pts',(-5.49440633438804,67.8605605910626,6.00000000000048));
#7696=CARTESIAN_POINT('Ctrl Pts',(-5.63943167744069,67.9383073892477,6.00000000000019));
#7697=CARTESIAN_POINT('Ctrl Pts',(-5.76042394103096,68.0031702670131,5.99999999999995));
#7698=CARTESIAN_POINT('Ctrl Pts',(-5.88061928742128,68.0702983394636,6.));
#7699=CARTESIAN_POINT('Ctrl Pts',(-5.99998978176463,68.1396964325479,6.));
#7700=CARTESIAN_POINT('',(-6.,16.9705627484771,6.));
#7701=CARTESIAN_POINT('',(-6.,68.1396788547224,6.));
#7702=CARTESIAN_POINT('',(-8.,14.8323969741913,6.));
#7703=CARTESIAN_POINT('Ctrl Pts',(-6.,16.9705627484771,6.));
#7704=CARTESIAN_POINT('Ctrl Pts',(-6.,16.7029092618308,6.));
#7705=CARTESIAN_POINT('Ctrl Pts',(-6.06020384677459,16.3874179356908,6.));
#7706=CARTESIAN_POINT('Ctrl Pts',(-6.25585405294364,15.8960743911704,6.));
#7707=CARTESIAN_POINT('Ctrl Pts',(-6.42385919064368,15.6314481148128,6.));
#7708=CARTESIAN_POINT('Ctrl Pts',(-6.7778910457933,15.2614647616422,6.));
#7709=CARTESIAN_POINT('Ctrl Pts',(-7.02372732242562,15.0877073947429,6.));
#7710=CARTESIAN_POINT('Ctrl Pts',(-7.47536381734142,14.8921163084765,6.));
#7711=CARTESIAN_POINT('Ctrl Pts',(-7.75869936772315,14.8323969741913,6.));
#7712=CARTESIAN_POINT('Ctrl Pts',(-8.,14.8323969741913,6.));
#7713=CARTESIAN_POINT('',(8.,14.8323969741913,6.));
#7714=CARTESIAN_POINT('',(8.,14.8323969741913,6.));
#7715=CARTESIAN_POINT('Ctrl Pts',(8.,14.8323969741913,6.));
#7716=CARTESIAN_POINT('Ctrl Pts',(7.75869936772315,14.8323969741913,6.));
#7717=CARTESIAN_POINT('Ctrl Pts',(7.47536381734142,14.8921163084765,6.));
#7718=CARTESIAN_POINT('Ctrl Pts',(7.02372732242562,15.0877073947429,6.));
#7719=CARTESIAN_POINT('Ctrl Pts',(6.7778910457933,15.2614647616422,6.));
#7720=CARTESIAN_POINT('Ctrl Pts',(6.42385919064368,15.6314481148128,6.));
#7721=CARTESIAN_POINT('Ctrl Pts',(6.25585405294364,15.8960743911704,6.));
#7722=CARTESIAN_POINT('Ctrl Pts',(6.06020384677459,16.3874179356908,6.));
#7723=CARTESIAN_POINT('Ctrl Pts',(6.,16.7029092618308,6.));
#7724=CARTESIAN_POINT('Ctrl Pts',(6.,16.9705627484771,6.));
#7725=CARTESIAN_POINT('Origin',(0.,0.,-6.));
#7726=CARTESIAN_POINT('',(-6.,68.1396788547224,-6.));
#7727=CARTESIAN_POINT('',(-6.,16.9705627484771,-6.));
#7728=CARTESIAN_POINT('',(-6.,68.1396788547224,-6.));
#7729=CARTESIAN_POINT('Ctrl Pts',(-6.00000000000001,68.1396788547224,-6.00000000033548));
#7730=CARTESIAN_POINT('Ctrl Pts',(-5.88135123476548,68.0707064539889,-6.00000000021859));
#7731=CARTESIAN_POINT('Ctrl Pts',(-5.76179150219477,68.0039433666279,-6.0000000001483));
#7732=CARTESIAN_POINT('Ctrl Pts',(-5.64128502565881,67.9393234853503,-6.00000000010555));
#7733=CARTESIAN_POINT('Ctrl Pts',(-5.35454183345322,67.7855615335439,-6.00000000000383));
#7734=CARTESIAN_POINT('Ctrl Pts',(-5.06243931289424,67.6439341165104,-5.99999999997568));
#7735=CARTESIAN_POINT('Ctrl Pts',(-4.7653752487817,67.51447477604,-6.00000000011691));
#7736=CARTESIAN_POINT('Ctrl Pts',(-4.70765521754892,67.4893206154462,-6.00000000014435));
#7737=CARTESIAN_POINT('Ctrl Pts',(-4.64974783530638,67.4646258594542,-6.00000000018246));
#7738=CARTESIAN_POINT('Ctrl Pts',(-4.59164625233319,67.440390106457,-6.00000000024038));
#7739=CARTESIAN_POINT('Ctrl Pts',(-4.35024698211367,67.3396958949164,-6.00000000048101));
#7740=CARTESIAN_POINT('Ctrl Pts',(-4.10557127976831,67.2469034855812,-6.00000000012488));
#7741=CARTESIAN_POINT('Ctrl Pts',(-3.857028682324,67.1619865543543,-6.00000000004164));
#7742=CARTESIAN_POINT('Ctrl Pts',(-3.85632817266295,67.1617472185973,-6.0000000000414));
#7743=CARTESIAN_POINT('Ctrl Pts',(-3.85562763231577,67.161507945473,-6.00000000004117));
#7744=CARTESIAN_POINT('Ctrl Pts',(-3.85492706127251,67.161268734981,-6.00000000004094));
#7745=CARTESIAN_POINT('Ctrl Pts',(-3.60706325630569,67.0766354585685,-5.9999999999591));
#7746=CARTESIAN_POINT('Ctrl Pts',(-3.35536071028375,66.9998438175543,-6.));
#7747=CARTESIAN_POINT('Ctrl Pts',(-3.10247303323778,66.9316279187809,-6.));
#7748=CARTESIAN_POINT('Ctrl Pts',(-3.03891432167408,66.9144830950993,-6.));
#7749=CARTESIAN_POINT('Ctrl Pts',(-2.97524844790974,66.8978716712467,-5.99999999999992));
#7750=CARTESIAN_POINT('Ctrl Pts',(-2.91151863585045,66.8818072455702,-6.00000000000031));
#7751=CARTESIAN_POINT('Ctrl Pts',(-2.63102181288571,66.8111021827525,-6.00000000000201));
#7752=CARTESIAN_POINT('Ctrl Pts',(-2.34928633703758,66.7509976829606,-6.0000000000383));
#7753=CARTESIAN_POINT('Ctrl Pts',(-2.06637325397113,66.7012185486804,-6.00000000006218));
#7754=CARTESIAN_POINT('Ctrl Pts',(-2.02907999731538,66.694656724071,-6.00000000006533));
#7755=CARTESIAN_POINT('Ctrl Pts',(-1.99176628159546,66.6882742410331,-6.00000000006784));
#7756=CARTESIAN_POINT('Ctrl Pts',(-1.95443224984977,66.6820704027054,-6.00000000006935));
#7757=CARTESIAN_POINT('Ctrl Pts',(-1.82582569506263,66.6606997058783,-6.00000000007455));
#7758=CARTESIAN_POINT('Ctrl Pts',(-1.69697805757653,66.6414490286518,-6.00000000006504));
#7759=CARTESIAN_POINT('Ctrl Pts',(-1.56792279424157,66.6243169437229,-6.00000000004334));
#7760=CARTESIAN_POINT('Ctrl Pts',(-1.37527749253196,66.5987432818299,-6.00000000001095));
#7761=CARTESIAN_POINT('Ctrl Pts',(-1.18208097804144,66.5778870888126,-6.00000000000977));
#7762=CARTESIAN_POINT('Ctrl Pts',(-0.988407256485119,66.5617481221748,-6.00000000000759));
#7763=CARTESIAN_POINT('Ctrl Pts',(-0.665022342205425,66.5348002311508,-6.00000000000395));
#7764=CARTESIAN_POINT('Ctrl Pts',(-0.340306945124361,66.5210055006354,-6.00000000000648));
#7765=CARTESIAN_POINT('Ctrl Pts',(-0.0134586100326744,66.5206838218603,
-6.00000000000188));
#7766=CARTESIAN_POINT('Ctrl Pts',(-0.0124519601418355,66.5206828311319,
-6.00000000000187));
#7767=CARTESIAN_POINT('Ctrl Pts',(-0.0114452900197199,66.5206819681829,
-6.00000000000185));
#7768=CARTESIAN_POINT('Ctrl Pts',(-0.0104385997885719,66.5206812330135,
-6.00000000000184));
#7769=CARTESIAN_POINT('Ctrl Pts',(0.251373358176787,66.5204900360357,-5.99999999999816));
#7770=CARTESIAN_POINT('Ctrl Pts',(0.514448035954128,66.5289433967365,-6.));
#7771=CARTESIAN_POINT('Ctrl Pts',(0.776872929457171,66.5460551200837,-6.));
#7772=CARTESIAN_POINT('Ctrl Pts',(0.84113945443676,66.5502456943134,-6.));
#7773=CARTESIAN_POINT('Ctrl Pts',(0.905383773332602,66.5549590297467,-5.99999999999899));
#7774=CARTESIAN_POINT('Ctrl Pts',(0.96956591794925,66.5601942307276,-6.0000000000062));
#7775=CARTESIAN_POINT('Ctrl Pts',(1.16746410942001,66.5763363651527,-6.00000000002842));
#7776=CARTESIAN_POINT('Ctrl Pts',(1.36476998969738,66.597443812802,-6.00000000018961));
#7777=CARTESIAN_POINT('Ctrl Pts',(1.56118391871842,66.6233966302541,-6.00000000007553));
#7778=CARTESIAN_POINT('Ctrl Pts',(1.68948047047876,66.6403488749558,-6.00000000000101));
#7779=CARTESIAN_POINT('Ctrl Pts',(1.81736883731735,66.6593790563258,-6.00000000000495));
#7780=CARTESIAN_POINT('Ctrl Pts',(1.94492176430178,66.6804804617521,-6.00000000000425));
#7781=CARTESIAN_POINT('Ctrl Pts',(2.07597587522071,66.7021610769498,-6.00000000000353));
#7782=CARTESIAN_POINT('Ctrl Pts',(2.20667590863535,66.7260281326416,-5.9999999999992));
#7783=CARTESIAN_POINT('Ctrl Pts',(2.33707867056231,66.7521088426973,-6.00000000006009));
#7784=CARTESIAN_POINT('Ctrl Pts',(2.52789038140951,66.7902714155777,-6.00000000014919));
#7785=CARTESIAN_POINT('Ctrl Pts',(2.71803095889827,66.8331402961369,-6.00000000004381));
#7786=CARTESIAN_POINT('Ctrl Pts',(2.90717461949266,66.8807206424077,-6.00000000001451));
#7787=CARTESIAN_POINT('Ctrl Pts',(2.97310322799981,66.897305422527,-6.0000000000043));
#7788=CARTESIAN_POINT('Ctrl Pts',(3.03891073048377,66.9144622409335,-6.0000000000018));
#7789=CARTESIAN_POINT('Ctrl Pts',(3.10455475004544,66.932177232458,-6.00000000000118));
#7790=CARTESIAN_POINT('Ctrl Pts',(3.30454500276501,66.9861475050824,-5.99999999999932));
#7791=CARTESIAN_POINT('Ctrl Pts',(3.50317683929644,67.045322334494,-5.99999999998744));
#7792=CARTESIAN_POINT('Ctrl Pts',(3.69973730005121,67.1094558520618,-6.00000000001292));
#7793=CARTESIAN_POINT('Ctrl Pts',(3.7500829322271,67.1258825661284,-6.00000000001944));
#7794=CARTESIAN_POINT('Ctrl Pts',(3.80029253777679,67.1426348178705,-6.00000000002988));
#7795=CARTESIAN_POINT('Ctrl Pts',(3.85035380604943,67.1597089272837,-6.00000000005043));
#7796=CARTESIAN_POINT('Ctrl Pts',(3.85304807262321,67.1606278453187,-6.00000000005154));
#7797=CARTESIAN_POINT('Ctrl Pts',(3.85574190949298,67.1615476956639,-6.00000000005268));
#7798=CARTESIAN_POINT('Ctrl Pts',(3.85843531784378,67.1624684786439,-6.00000000005384));
#7799=CARTESIAN_POINT('Ctrl Pts',(4.10656203133196,67.247294403611,-6.00000000016149));
#7800=CARTESIAN_POINT('Ctrl Pts',(4.35103204358516,67.3400159519093,-6.00000000044336));
#7801=CARTESIAN_POINT('Ctrl Pts',(4.5922509791071,67.4406456432544,-6.00000000022157));
#7802=CARTESIAN_POINT('Ctrl Pts',(4.64834046407308,67.4640445839206,-6.00000000016999));
#7803=CARTESIAN_POINT('Ctrl Pts',(4.70424963404129,67.4878714386743,-6.00000000013519));
#7804=CARTESIAN_POINT('Ctrl Pts',(4.75998502568673,67.5121269723368,-6.00000000010976));
#7805=CARTESIAN_POINT('Ctrl Pts',(5.05700416524726,67.6413869905284,-5.99999999997425));
#7806=CARTESIAN_POINT('Ctrl Pts',(5.34908932208966,67.7828195726981,-6.00000000000132));
#7807=CARTESIAN_POINT('Ctrl Pts',(5.63593680564189,67.9364541673593,-6.00000000008223));
#7808=CARTESIAN_POINT('Ctrl Pts',(5.75823770305734,68.0019581368152,-6.00000000011673));
#7809=CARTESIAN_POINT('Ctrl Pts',(5.879586265764,68.0696804496391,-6.00000000017492));
#7810=CARTESIAN_POINT('Ctrl Pts',(5.99999999999993,68.1396788547225,-6.00000000027673));
#7811=CARTESIAN_POINT('',(8.,14.8323969741913,-6.));
#7812=CARTESIAN_POINT('Ctrl Pts',(6.,16.9705627484771,-6.));
#7813=CARTESIAN_POINT('Ctrl Pts',(6.,16.7029092618308,-6.));
#7814=CARTESIAN_POINT('Ctrl Pts',(6.06020384677459,16.3874179356908,-6.));
#7815=CARTESIAN_POINT('Ctrl Pts',(6.25585405294364,15.8960743911704,-6.));
#7816=CARTESIAN_POINT('Ctrl Pts',(6.42385919064368,15.6314481148128,-6.));
#7817=CARTESIAN_POINT('Ctrl Pts',(6.7778910457933,15.2614647616422,-6.));
#7818=CARTESIAN_POINT('Ctrl Pts',(7.02372732242562,15.0877073947429,-6.));
#7819=CARTESIAN_POINT('Ctrl Pts',(7.47536381734142,14.8921163084765,-6.));
#7820=CARTESIAN_POINT('Ctrl Pts',(7.75869936772315,14.8323969741913,-6.));
#7821=CARTESIAN_POINT('Ctrl Pts',(8.,14.8323969741913,-6.));
#7822=CARTESIAN_POINT('',(-8.,14.8323969741913,-6.));
#7823=CARTESIAN_POINT('',(8.,14.8323969741913,-6.));
#7824=CARTESIAN_POINT('Ctrl Pts',(-8.,14.8323969741913,-6.));
#7825=CARTESIAN_POINT('Ctrl Pts',(-7.75869936772315,14.8323969741913,-6.));
#7826=CARTESIAN_POINT('Ctrl Pts',(-7.47536381734142,14.8921163084765,-6.));
#7827=CARTESIAN_POINT('Ctrl Pts',(-7.02372732242562,15.0877073947429,-6.));
#7828=CARTESIAN_POINT('Ctrl Pts',(-6.7778910457933,15.2614647616422,-6.));
#7829=CARTESIAN_POINT('Ctrl Pts',(-6.42385919064368,15.6314481148128,-6.));
#7830=CARTESIAN_POINT('Ctrl Pts',(-6.25585405294364,15.8960743911704,-6.));
#7831=CARTESIAN_POINT('Ctrl Pts',(-6.06020384677459,16.3874179356908,-6.));
#7832=CARTESIAN_POINT('Ctrl Pts',(-6.,16.7029092618308,-6.));
#7833=CARTESIAN_POINT('Ctrl Pts',(-6.,16.9705627484771,-6.));
#7834=CARTESIAN_POINT('Origin',(0.,6.,-2.09488880330588E-14));
#7835=CARTESIAN_POINT('Ctrl Pts',(6.00000000000008,6.00000000309571,-68.1396788547223));
#7836=CARTESIAN_POINT('Ctrl Pts',(5.88443053952251,6.00000000152898,-68.0725017211956));
#7837=CARTESIAN_POINT('Ctrl Pts',(5.76781164854468,6.00000000116511,-68.0073271284604));
#7838=CARTESIAN_POINT('Ctrl Pts',(5.65007008364704,6.00000000095536,-67.9440866077606));
#7839=CARTESIAN_POINT('Ctrl Pts',(5.47466763156413,6.0000000006429,-67.8498756771399));
#7840=CARTESIAN_POINT('Ctrl Pts',(5.29677696751753,6.000000000858,-67.7599563862543));
#7841=CARTESIAN_POINT('Ctrl Pts',(5.11705077455563,6.00000000100214,-67.6746189934296));
#7842=CARTESIAN_POINT('Ctrl Pts',(5.00046956793888,6.00000000109564,-67.6192640334147));
#7843=CARTESIAN_POINT('Ctrl Pts',(4.88311488344197,6.00000000115652,-67.565837369108));
#7844=CARTESIAN_POINT('Ctrl Pts',(4.76515531729687,6.00000000101204,-67.5144247705252));
#7845=CARTESIAN_POINT('Ctrl Pts',(4.70524037260182,6.00000000093865,-67.4883108816615));
#7846=CARTESIAN_POINT('Ctrl Pts',(4.64516926942165,6.00000000081218,-67.4627166925166));
#7847=CARTESIAN_POINT('Ctrl Pts',(4.58494545881954,6.0000000006505,-67.4376372856515));
#7848=CARTESIAN_POINT('Ctrl Pts',(4.34284135212469,6.00000000000053,-67.3368162426988));
#7849=CARTESIAN_POINT('Ctrl Pts',(4.0981160083979,6.00000000028404,-67.2443422503418));
#7850=CARTESIAN_POINT('Ctrl Pts',(3.85139338320861,6.00000000163487,-67.1601340992298));
#7851=CARTESIAN_POINT('Ctrl Pts',(3.60459794198451,6.0000000029861,-67.0759010954977));
#7852=CARTESIAN_POINT('Ctrl Pts',(3.35580404208615,6.00000000623266,-66.9999387113475));
#7853=CARTESIAN_POINT('Ctrl Pts',(3.10471881286491,6.00000000804558,-66.9321924190084));
#7854=CARTESIAN_POINT('Ctrl Pts',(2.86855020564974,6.0000000097508,-66.8684708390678));
#7855=CARTESIAN_POINT('Ctrl Pts',(2.63069277643225,6.00000000585791,-66.8120699357947));
#7856=CARTESIAN_POINT('Ctrl Pts',(2.39076110075127,6.00000000323229,-66.7629601317855));
#7857=CARTESIAN_POINT('Ctrl Pts',(2.24875049531973,6.00000000167824,-66.7338930526673));
#7858=CARTESIAN_POINT('Ctrl Pts',(2.10601323548916,6.00000000066935,-66.7073812094719));
#7859=CARTESIAN_POINT('Ctrl Pts',(1.96246914678003,6.00000000028938,-66.6834270406419));
#7860=CARTESIAN_POINT('Ctrl Pts',(1.83293087812574,5.9999999999465,-66.6618101173314));
#7861=CARTESIAN_POINT('Ctrl Pts',(1.70273547973188,5.99999999999977,-66.6422761731934));
#7862=CARTESIAN_POINT('Ctrl Pts',(1.5720255845334,5.99999999999977,-66.6248804795373));
#7863=CARTESIAN_POINT('Ctrl Pts',(1.40616078506809,5.99999999999977,-66.6028061504634));
#7864=CARTESIAN_POINT('Ctrl Pts',(1.23927157998101,6.00000000003217,-66.5841437759783));
#7865=CARTESIAN_POINT('Ctrl Pts',(1.07202619547598,6.0000000000765,-66.5690240649954));
#7866=CARTESIAN_POINT('Ctrl Pts',(1.04376272367814,6.00000000008399,-66.5664689240794));
#7867=CARTESIAN_POINT('Ctrl Pts',(1.01548909646327,6.00000000009016,-66.5640148386483));
#7868=CARTESIAN_POINT('Ctrl Pts',(0.987208553067123,6.00000000009342,-66.5616622922949));
#7869=CARTESIAN_POINT('Ctrl Pts',(0.920377643541939,6.00000000010111,-66.5561028937254));
#7870=CARTESIAN_POINT('Ctrl Pts',(0.853508114226926,6.0000000000884,-66.5511106251358));
#7871=CARTESIAN_POINT('Ctrl Pts',(0.786635623670159,6.00000000005849,-66.546683494606));
#7872=CARTESIAN_POINT('Ctrl Pts',(0.595551811466195,5.99999999997304,-66.5340332557451));
#7873=CARTESIAN_POINT('Ctrl Pts',(0.404475822382095,5.99999999999819,-66.5260266785561));
#7874=CARTESIAN_POINT('Ctrl Pts',(0.213506141043386,6.00000000000357,-66.5226020043316));
#7875=CARTESIAN_POINT('Ctrl Pts',(0.143592221144975,6.00000000000553,-66.5213482325406));
#7876=CARTESIAN_POINT('Ctrl Pts',(0.0736925003305599,6.00000000000947,-66.520709072491));
#7877=CARTESIAN_POINT('Ctrl Pts',(0.00381174273192314,6.00000000002068,
-66.5206832338361));
#7878=CARTESIAN_POINT('Ctrl Pts',(0.00223179946017313,6.00000000002093,
-66.5206826496465));
#7879=CARTESIAN_POINT('Ctrl Pts',(0.000651865883589953,6.00000000002119,
-66.5206823790097));
#7880=CARTESIAN_POINT('Ctrl Pts',(-0.000928058234337155,6.00000000002145,
-66.5206824219519));
#7881=CARTESIAN_POINT('Ctrl Pts',(-0.263264677338428,6.00000000006482,-66.520689552242));
#7882=CARTESIAN_POINT('Ctrl Pts',(-0.525331339169259,6.00000000028711,-66.5293351560878));
#7883=CARTESIAN_POINT('Ctrl Pts',(-0.787710887408489,6.00000000019101,-66.5467414956877));
#7884=CARTESIAN_POINT('Ctrl Pts',(-0.851266591343311,6.00000000016774,-66.5509578005545));
#7885=CARTESIAN_POINT('Ctrl Pts',(-0.914818365061761,6.00000000013568,-66.5556874880789));
#7886=CARTESIAN_POINT('Ctrl Pts',(-0.978365706981233,6.00000000010664,-66.560931726518));
#7887=CARTESIAN_POINT('Ctrl Pts',(-1.17716339205941,6.00000000001582,-66.5773374868567));
#7888=CARTESIAN_POINT('Ctrl Pts',(-1.37591689807605,5.99999999999977,-66.5987815572106));
#7889=CARTESIAN_POINT('Ctrl Pts',(-1.57344188122075,5.99999999999977,-66.6250804427651));
#7890=CARTESIAN_POINT('Ctrl Pts',(-1.70144110734177,5.99999999999977,-66.6421225249627));
#7891=CARTESIAN_POINT('Ctrl Pts',(-1.82903601209464,5.99999999999399,-66.6612185682778));
#7892=CARTESIAN_POINT('Ctrl Pts',(-1.95599749600092,6.0000000000624,-66.6823299049636));
#7893=CARTESIAN_POINT('Ctrl Pts',(-2.08758818528542,6.0000000001333,-66.7042109925243));
#7894=CARTESIAN_POINT('Ctrl Pts',(-2.21849837114969,6.00000000030333,-66.7282569777027));
#7895=CARTESIAN_POINT('Ctrl Pts',(-2.34882467025348,6.00000000042092,-66.7544592401104));
#7896=CARTESIAN_POINT('Ctrl Pts',(-2.53816635487132,6.00000000059176,-66.7925266182157));
#7897=CARTESIAN_POINT('Ctrl Pts',(-2.72608639026754,6.00000000028953,-66.8350974685097));
#7898=CARTESIAN_POINT('Ctrl Pts',(-2.91266554092604,6.00000000015476,-66.8821207250386));
#7899=CARTESIAN_POINT('Ctrl Pts',(-2.97841818014486,6.00000000010727,-66.8986922616252));
#7900=CARTESIAN_POINT('Ctrl Pts',(-3.04400427898507,6.00000000007635,-66.9158166284133));
#7901=CARTESIAN_POINT('Ctrl Pts',(-3.10941746042439,6.00000000006051,-66.933492240734));
#7902=CARTESIAN_POINT('Ctrl Pts',(-3.35744519690348,6.00000000000045,-67.0005130157267));
#7903=CARTESIAN_POINT('Ctrl Pts',(-3.60321039549219,6.00000000000121,-67.0755019333164));
#7904=CARTESIAN_POINT('Ctrl Pts',(-3.84653444986901,6.00000000001263,-67.1583991671131));
#7905=CARTESIAN_POINT('Ctrl Pts',(-4.09574737289984,6.00000000002432,-67.2433026592835));
#7906=CARTESIAN_POINT('Ctrl Pts',(-4.34239946517691,5.99999999999479,-67.336501827309));
#7907=CARTESIAN_POINT('Ctrl Pts',(-4.58683540182128,6.00000000045564,-67.4383837794248));
#7908=CARTESIAN_POINT('Ctrl Pts',(-4.64389967612715,6.00000000056323,-67.4621684149501));
#7909=CARTESIAN_POINT('Ctrl Pts',(-4.70081907510701,6.00000000064926,-67.4864135837856));
#7910=CARTESIAN_POINT('Ctrl Pts',(-4.75761051430218,6.00000000070297,-67.5111290206764));
#7911=CARTESIAN_POINT('Ctrl Pts',(-4.91645120347176,6.00000000085317,-67.5802559363611));
#7912=CARTESIAN_POINT('Ctrl Pts',(-5.07429236532074,6.00000000074464,-67.6530582185577));
#7913=CARTESIAN_POINT('Ctrl Pts',(-5.23069101215385,6.00000000068362,-67.7293290427591));
#7914=CARTESIAN_POINT('Ctrl Pts',(-5.36954056109083,6.00000000062944,-67.7970417100477));
#7915=CARTESIAN_POINT('Ctrl Pts',(-5.50725375393251,6.00000000059421,-67.8674892809091));
#7916=CARTESIAN_POINT('Ctrl Pts',(-5.6434987472227,6.00000000084558,-67.9405537264822));
#7917=CARTESIAN_POINT('Ctrl Pts',(-5.76343389597552,6.00000000106685,-68.0048716506622));
#7918=CARTESIAN_POINT('Ctrl Pts',(-5.88223041979097,6.00000000143562,-68.0712175381268));
#7919=CARTESIAN_POINT('Ctrl Pts',(-6.00000000000007,6.00000000292373,-68.1396788547223));
#7920=CARTESIAN_POINT('',(-8.,5.99999999999995,-14.8323969741913));
#7921=CARTESIAN_POINT('Ctrl Pts',(-6.,5.99999999999994,-16.9705627484772));
#7922=CARTESIAN_POINT('Ctrl Pts',(-6.,5.99999999999994,-16.7029092618309));
#7923=CARTESIAN_POINT('Ctrl Pts',(-6.06020384677459,5.99999999999994,-16.3874179356908));
#7924=CARTESIAN_POINT('Ctrl Pts',(-6.25585405294364,5.99999999999994,-15.8960743911704));
#7925=CARTESIAN_POINT('Ctrl Pts',(-6.42385919064368,5.99999999999994,-15.6314481148128));
#7926=CARTESIAN_POINT('Ctrl Pts',(-6.7778910457933,5.99999999999995,-15.2614647616422));
#7927=CARTESIAN_POINT('Ctrl Pts',(-7.02372732242562,5.99999999999995,-15.0877073947429));
#7928=CARTESIAN_POINT('Ctrl Pts',(-7.47536381734142,5.99999999999995,-14.8921163084765));
#7929=CARTESIAN_POINT('Ctrl Pts',(-7.75869936772315,5.99999999999995,-14.8323969741913));
#7930=CARTESIAN_POINT('Ctrl Pts',(-8.,5.99999999999995,-14.8323969741913));
#7931=CARTESIAN_POINT('',(8.,5.99999999999995,-14.8323969741913));
#7932=CARTESIAN_POINT('',(8.,5.99999999999995,-14.8323969741913));
#7933=CARTESIAN_POINT('Ctrl Pts',(8.,5.99999999999995,-14.8323969741913));
#7934=CARTESIAN_POINT('Ctrl Pts',(7.75869936772315,5.99999999999995,-14.8323969741913));
#7935=CARTESIAN_POINT('Ctrl Pts',(7.47536381734142,5.99999999999995,-14.8921163084765));
#7936=CARTESIAN_POINT('Ctrl Pts',(7.02372732242562,5.99999999999995,-15.0877073947429));
#7937=CARTESIAN_POINT('Ctrl Pts',(6.7778910457933,5.99999999999995,-15.2614647616422));
#7938=CARTESIAN_POINT('Ctrl Pts',(6.42385919064368,5.99999999999994,-15.6314481148128));
#7939=CARTESIAN_POINT('Ctrl Pts',(6.25585405294364,5.99999999999994,-15.8960743911704));
#7940=CARTESIAN_POINT('Ctrl Pts',(6.06020384677459,5.99999999999994,-16.3874179356908));
#7941=CARTESIAN_POINT('Ctrl Pts',(6.,5.99999999999994,-16.7029092618309));
#7942=CARTESIAN_POINT('Ctrl Pts',(6.,5.99999999999994,-16.9705627484772));
#7943=CARTESIAN_POINT('Origin',(0.,-6.,2.09488880330588E-14));
#7944=CARTESIAN_POINT('Ctrl Pts',(-5.99997872967542,-6.00000000000024,-68.1397154447039));
#7945=CARTESIAN_POINT('Ctrl Pts',(-5.88065306094768,-6.00000000000024,-68.070356028456));
#7946=CARTESIAN_POINT('Ctrl Pts',(-5.76035179595835,-5.99999999978724,-68.0032029450616));
#7947=CARTESIAN_POINT('Ctrl Pts',(-5.63919789927778,-6.00000000114149,-67.938257741962));
#7948=CARTESIAN_POINT('Ctrl Pts',(-5.36452811515037,-6.00000000421175,-67.7910195151757));
#7949=CARTESIAN_POINT('Ctrl Pts',(-5.08547906226534,-6.00000002415142,-67.6551300980379));
#7950=CARTESIAN_POINT('Ctrl Pts',(-4.80172154724994,-6.00000003249791,-67.5303613497886));
#7951=CARTESIAN_POINT('Ctrl Pts',(-4.73247230274036,-6.00000003453481,-67.499912318142));
#7952=CARTESIAN_POINT('Ctrl Pts',(-4.66294239805607,-6.00000003545488,-67.4701255521591));
#7953=CARTESIAN_POINT('Ctrl Pts',(-4.59312657863782,-6.00000003465391,-67.4409976541893));
#7954=CARTESIAN_POINT('Ctrl Pts',(-4.39454299406212,-6.00000003237562,-67.358146483234));
#7955=CARTESIAN_POINT('Ctrl Pts',(-4.19396786917798,-6.00000002041265,-67.2807776472526));
#7956=CARTESIAN_POINT('Ctrl Pts',(-3.99105655262234,-6.00000001234683,-67.2087977787802));
#7957=CARTESIAN_POINT('Ctrl Pts',(-3.94543987688706,-6.00000001053355,-67.1926159197528));
#7958=CARTESIAN_POINT('Ctrl Pts',(-3.89970508733666,-6.00000000888316,-67.1767066229859));
#7959=CARTESIAN_POINT('Ctrl Pts',(-3.85384819076817,-6.0000000074552,-67.1610691807499));
#7960=CARTESIAN_POINT('Ctrl Pts',(-3.64869141653897,-6.00000000106674,-67.0911096447497));
#7961=CARTESIAN_POINT('Ctrl Pts',(-3.44109171841246,-6.00000000007894,-67.0265873650583));
#7962=CARTESIAN_POINT('Ctrl Pts',(-3.23159036684668,-6.00000000001056,-66.9676682583467));
#7963=CARTESIAN_POINT('Ctrl Pts',(-3.19055146412293,-5.99999999999717,-66.9561266836942));
#7964=CARTESIAN_POINT('Ctrl Pts',(-3.14943955853333,-6.00000000000023,-66.9448002727395));
#7965=CARTESIAN_POINT('Ctrl Pts',(-3.10825868593511,-6.00000000000023,-66.9336905046549));
#7966=CARTESIAN_POINT('Ctrl Pts',(-2.95466816752725,-6.00000000000023,-66.8922548834103));
#7967=CARTESIAN_POINT('Ctrl Pts',(-2.79997518606765,-6.00000000000023,-66.8537662550196));
#7968=CARTESIAN_POINT('Ctrl Pts',(-2.6448032490687,-6.00000000000023,-66.8183882438221));
#7969=CARTESIAN_POINT('Ctrl Pts',(-2.54365437995968,-6.00000000000023,-66.7953270776527));
#7970=CARTESIAN_POINT('Ctrl Pts',(-2.4423023734785,-6.00000000000023,-66.7735866407805));
#7971=CARTESIAN_POINT('Ctrl Pts',(-2.34092187223618,-6.00000000000023,-66.7532004707004));
#7972=CARTESIAN_POINT('Ctrl Pts',(-2.21137469343365,-6.00000000000023,-66.7271503842626));
#7973=CARTESIAN_POINT('Ctrl Pts',(-2.08172507159667,-5.99999999964996,-66.7033287187243));
#7974=CARTESIAN_POINT('Ctrl Pts',(-1.95199939961633,-6.00000000156985,-66.6817296203148));
#7975=CARTESIAN_POINT('Ctrl Pts',(-1.824463314101,-6.00000000345734,-66.6604950842376));
#7976=CARTESIAN_POINT('Ctrl Pts',(-1.69685357491418,-6.00000000797633,-66.6414087341013));
#7977=CARTESIAN_POINT('Ctrl Pts',(-1.56900071732305,-6.00000001702602,-66.6244302686289));
#7978=CARTESIAN_POINT('Ctrl Pts',(-1.33655492556664,-6.00000003347902,-66.5935621838328));
#7979=CARTESIAN_POINT('Ctrl Pts',(-1.10349609256449,-6.00000003523112,-66.5695462510003));
#7980=CARTESIAN_POINT('Ctrl Pts',(-0.869853272257425,-6.00000002613846,
-66.5524429803587));
#7981=CARTESIAN_POINT('Ctrl Pts',(-0.639795826763875,-6.00000001718533,
-66.5356021686093));
#7982=CARTESIAN_POINT('Ctrl Pts',(-0.409172035298845,-6.00000000564921,
-66.5254634964283));
#7983=CARTESIAN_POINT('Ctrl Pts',(-0.178031919006002,-6.00000000232865,
-66.5220391591688));
#7984=CARTESIAN_POINT('Ctrl Pts',(-0.123016782862887,-6.00000000153831,
-66.521224110775));
#7985=CARTESIAN_POINT('Ctrl Pts',(-0.0679725019716026,-6.00000000104546,
-66.5207892356362));
#7986=CARTESIAN_POINT('Ctrl Pts',(-0.0128999542220165,-6.00000000073503,
-66.5207343095857));
#7987=CARTESIAN_POINT('Ctrl Pts',(-0.012482287975762,-6.00000000073268,
-66.5207338930305));
#7988=CARTESIAN_POINT('Ctrl Pts',(-0.0120646200720832,-6.00000000073033,
-66.5207334982936));
#7989=CARTESIAN_POINT('Ctrl Pts',(-0.0116469505067236,-6.000000000728,-66.5207331253744));
#7990=CARTESIAN_POINT('Ctrl Pts',(0.169989366969348,-5.99999999971235,-66.5205709501121));
#7991=CARTESIAN_POINT('Ctrl Pts',(0.351939413797874,-6.00000000000218,-66.5245306974));
#7992=CARTESIAN_POINT('Ctrl Pts',(0.534215007419024,-6.00000000002061,-66.5326993242846));
#7993=CARTESIAN_POINT('Ctrl Pts',(0.613160572127682,-6.00000000002859,-66.5362372464468));
#7994=CARTESIAN_POINT('Ctrl Pts',(0.692167277879461,-6.00000000004884,-66.5405653421137));
#7995=CARTESIAN_POINT('Ctrl Pts',(0.771236245526539,-6.00000000012279,-66.5456937235993));
#7996=CARTESIAN_POINT('Ctrl Pts',(0.836809062903187,-6.00000000018411,-66.5499467501988));
#7997=CARTESIAN_POINT('Ctrl Pts',(0.902416572517938,-6.00000000023104,-66.5547456408318));
#7998=CARTESIAN_POINT('Ctrl Pts',(0.96802849280209,-6.00000000024428,-66.5600951583082));
#7999=CARTESIAN_POINT('Ctrl Pts',(1.13715461784052,-6.00000000027841,-66.5738844691179));
#8000=CARTESIAN_POINT('Ctrl Pts',(1.3063098085867,-6.00000000012487,-66.5913360753138));
#8001=CARTESIAN_POINT('Ctrl Pts',(1.47473506099623,-6.00000000007166,-66.6123416933938));
#8002=CARTESIAN_POINT('Ctrl Pts',(1.50208873361841,-6.00000000006302,-66.6157531818254));
#8003=CARTESIAN_POINT('Ctrl Pts',(1.52942316435998,-6.00000000005606,-66.6192583016056));
#8004=CARTESIAN_POINT('Ctrl Pts',(1.55673512158337,-6.00000000005077,-66.6228564609117));
#8005=CARTESIAN_POINT('Ctrl Pts',(1.68662492850993,-6.00000000002558,-66.6399685343434));
#8006=CARTESIAN_POINT('Ctrl Pts',(1.81617214090643,-6.0000000000153,-66.6592036204614));
#8007=CARTESIAN_POINT('Ctrl Pts',(1.94516884575325,-6.00000000000929,-66.6805232592598));
#8008=CARTESIAN_POINT('Ctrl Pts',(2.26860782880832,-5.99999999999422,-66.7339789060551));
#8009=CARTESIAN_POINT('Ctrl Pts',(2.58858611930201,-6.00000000000024,-66.8005396713465));
#8010=CARTESIAN_POINT('Ctrl Pts',(2.9066523490031,-6.00000000000024,-66.8805814871616));
#8011=CARTESIAN_POINT('Ctrl Pts',(2.97098604581056,-6.00000000000024,-66.8967711528026));
#8012=CARTESIAN_POINT('Ctrl Pts',(3.0352415115127,-6.00000000000024,-66.9135123439025));
#8013=CARTESIAN_POINT('Ctrl Pts',(3.0993837879325,-6.00000000000024,-66.9307945087936));
#8014=CARTESIAN_POINT('Ctrl Pts',(3.35209374305792,-6.00000000000024,-66.9988833786916));
#8015=CARTESIAN_POINT('Ctrl Pts',(3.60338827102687,-5.99999999998588,-67.0754603115548));
#8016=CARTESIAN_POINT('Ctrl Pts',(3.85114437890632,-6.0000000000146,-67.159971681504));
#8017=CARTESIAN_POINT('Ctrl Pts',(3.85228098497779,-6.00000000001474,-67.1603593859163));
#8018=CARTESIAN_POINT('Ctrl Pts',(3.85341751650643,-6.00000000001487,-67.1607472573209));
#8019=CARTESIAN_POINT('Ctrl Pts',(3.85455397349793,-6.000000000015,-67.1611352957054));
#8020=CARTESIAN_POINT('Ctrl Pts',(4.10341404208677,-6.00000000004453,-67.2461075029162));
#8021=CARTESIAN_POINT('Ctrl Pts',(4.34869348585104,-6.00000000022622,-67.3390831996519));
#8022=CARTESIAN_POINT('Ctrl Pts',(4.59052929362912,-6.00000000011317,-67.4399236158872));
#8023=CARTESIAN_POINT('Ctrl Pts',(4.6483342431954,-6.00000000008615,-67.464027057095));
#8024=CARTESIAN_POINT('Ctrl Pts',(4.70594363997126,-6.00000000006834,-67.4885826241901));
#8025=CARTESIAN_POINT('Ctrl Pts',(4.763357441056,-6.0000000000555,-67.513588419992));
#8026=CARTESIAN_POINT('Ctrl Pts',(5.06065596138665,-5.99999999998898,-67.6430727243079));
#8027=CARTESIAN_POINT('Ctrl Pts',(5.35270991438456,-6.00000000000393,-67.7846295793901));
#8028=CARTESIAN_POINT('Ctrl Pts',(5.63934396309719,-6.00000000004665,-67.9382748405765));
#8029=CARTESIAN_POINT('Ctrl Pts',(5.76052186835046,-6.0000000000647,-68.0032301764352));
#8030=CARTESIAN_POINT('Ctrl Pts',(5.8807310423892,-6.00000000009423,-68.0703459263676));
#8031=CARTESIAN_POINT('Ctrl Pts',(5.99999999999997,-6.00000000014129,-68.1396788547224));
#8032=CARTESIAN_POINT('',(8.,-6.00000000000005,-14.8323969741913));
#8033=CARTESIAN_POINT('Ctrl Pts',(6.,-6.00000000000006,-16.9705627484771));
#8034=CARTESIAN_POINT('Ctrl Pts',(6.,-6.00000000000006,-16.7029092618308));
#8035=CARTESIAN_POINT('Ctrl Pts',(6.06020384677459,-6.00000000000006,-16.3874179356908));
#8036=CARTESIAN_POINT('Ctrl Pts',(6.25585405294365,-6.00000000000006,-15.8960743911704));
#8037=CARTESIAN_POINT('Ctrl Pts',(6.42385919064368,-6.00000000000006,-15.6314481148128));
#8038=CARTESIAN_POINT('Ctrl Pts',(6.7778910457933,-6.00000000000005,-15.2614647616422));
#8039=CARTESIAN_POINT('Ctrl Pts',(7.02372732242562,-6.00000000000005,-15.0877073947429));
#8040=CARTESIAN_POINT('Ctrl Pts',(7.47536381734142,-6.00000000000005,-14.8921163084765));
#8041=CARTESIAN_POINT('Ctrl Pts',(7.75869936772315,-6.00000000000005,-14.8323969741913));
#8042=CARTESIAN_POINT('Ctrl Pts',(8.,-6.00000000000005,-14.8323969741913));
#8043=CARTESIAN_POINT('',(-8.,-6.00000000000005,-14.8323969741913));
#8044=CARTESIAN_POINT('',(8.,-6.00000000000005,-14.8323969741913));
#8045=CARTESIAN_POINT('Ctrl Pts',(-8.,-6.00000000000005,-14.8323969741913));
#8046=CARTESIAN_POINT('Ctrl Pts',(-7.75869936772315,-6.00000000000005,-14.8323969741913));
#8047=CARTESIAN_POINT('Ctrl Pts',(-7.47536381734142,-6.00000000000005,-14.8921163084765));
#8048=CARTESIAN_POINT('Ctrl Pts',(-7.02372732242562,-6.00000000000005,-15.0877073947429));
#8049=CARTESIAN_POINT('Ctrl Pts',(-6.7778910457933,-6.00000000000005,-15.2614647616422));
#8050=CARTESIAN_POINT('Ctrl Pts',(-6.42385919064368,-6.00000000000006,-15.6314481148128));
#8051=CARTESIAN_POINT('Ctrl Pts',(-6.25585405294364,-6.00000000000006,-15.8960743911704));
#8052=CARTESIAN_POINT('Ctrl Pts',(-6.06020384677459,-6.00000000000006,-16.3874179356908));
#8053=CARTESIAN_POINT('Ctrl Pts',(-6.,-6.00000000000006,-16.7029092618308));
#8054=CARTESIAN_POINT('Ctrl Pts',(-6.,-6.00000000000006,-16.9705627484771));
#8055=CARTESIAN_POINT('Origin',(0.,6.,-2.09488880330588E-14));
#8056=CARTESIAN_POINT('',(5.99999160300743,6.00000000000024,68.1397295132015));
#8057=CARTESIAN_POINT('Ctrl Pts',(-5.99999999999999,6.00000000023105,68.1396788547224));
#8058=CARTESIAN_POINT('Ctrl Pts',(-5.88444358312955,6.00000000011434,68.0725115980034));
#8059=CARTESIAN_POINT('Ctrl Pts',(-5.76789237998722,6.00000000006755,68.0073544868762));
#8060=CARTESIAN_POINT('Ctrl Pts',(-5.65036932229242,6.00000000004037,67.9441916161475));
#8061=CARTESIAN_POINT('Ctrl Pts',(-5.3873288140795,5.99999999997953,67.8028202636442));
#8062=CARTESIAN_POINT('Ctrl Pts',(-5.1194177726107,6.0000000000003,67.6714423841422));
#8063=CARTESIAN_POINT('Ctrl Pts',(-4.84664783679216,6.00000000000025,67.5502106840568));
#8064=CARTESIAN_POINT('Ctrl Pts',(-4.82125130085735,6.00000000000024,67.5389232772595));
#8065=CARTESIAN_POINT('Ctrl Pts',(-4.79581266378767,6.00000000000024,67.5277237930512));
#8066=CARTESIAN_POINT('Ctrl Pts',(-4.77033194696672,6.00000000000024,67.5166123348889));
#8067=CARTESIAN_POINT('Ctrl Pts',(-4.70876721194481,6.00000000000023,67.4897656028181));
#8068=CARTESIAN_POINT('Ctrl Pts',(-4.64695686427904,6.00000000000024,67.463432758374));
#8069=CARTESIAN_POINT('Ctrl Pts',(-4.5849461772848,6.00000000000024,67.4376274899832));
#8070=CARTESIAN_POINT('Ctrl Pts',(-4.38827148386229,6.00000000000024,67.3557828355303));
#8071=CARTESIAN_POINT('Ctrl Pts',(-4.18925929943197,5.9999999999863,67.2791062947266));
#8072=CARTESIAN_POINT('Ctrl Pts',(-3.98903483489981,6.00000000001416,67.2080000447656));
#8073=CARTESIAN_POINT('Ctrl Pts',(-3.94362722082296,6.00000000002047,67.1918743172517));
#8074=CARTESIAN_POINT('Ctrl Pts',(-3.8981571587602,6.00000000003015,67.1760352619909));
#8075=CARTESIAN_POINT('Ctrl Pts',(-3.85263764092992,6.00000000004771,67.1604879161245));
#8076=CARTESIAN_POINT('Ctrl Pts',(-3.85062837020849,6.00000000004849,67.1598016428876));
#8077=CARTESIAN_POINT('Ctrl Pts',(-3.84861900312364,6.00000000004928,67.1591159380443));
#8078=CARTESIAN_POINT('Ctrl Pts',(-3.84660953923603,6.00000000005009,67.1584308013561));
#8079=CARTESIAN_POINT('Ctrl Pts',(-3.59833898175711,6.00000000014983,67.0737817222825));
#8080=CARTESIAN_POINT('Ctrl Pts',(-3.34861996632779,6.00000000048239,66.9978044385423));
#8081=CARTESIAN_POINT('Ctrl Pts',(-3.0970540533494,6.00000000024139,66.9301379860738));
#8082=CARTESIAN_POINT('Ctrl Pts',(-3.03681722293726,6.00000000018369,66.9139354228025));
#8083=CARTESIAN_POINT('Ctrl Pts',(-2.97647791034341,6.00000000014616,66.8982129891066));
#8084=CARTESIAN_POINT('Ctrl Pts',(-2.91603033355864,6.00000000011925,66.8829659566196));
#8085=CARTESIAN_POINT('Ctrl Pts',(-2.60112596601868,5.99999999997907,66.8035358557358));
#8086=CARTESIAN_POINT('Ctrl Pts',(-2.28328401837121,6.00000000001375,66.7370060636242));
#8087=CARTESIAN_POINT('Ctrl Pts',(-1.96277620531409,6.00000000011972,66.6834659686194));
#8088=CARTESIAN_POINT('Ctrl Pts',(-1.83093099886256,6.00000000016332,66.6614415293022));
#8089=CARTESIAN_POINT('Ctrl Pts',(-1.69863458891165,6.00000000023189,66.6416154643382));
#8090=CARTESIAN_POINT('Ctrl Pts',(-1.56583784127881,6.00000000033247,66.6240105759369));
#8091=CARTESIAN_POINT('Ctrl Pts',(-1.37578755107881,6.0000000004764,66.5988155752367));
#8092=CARTESIAN_POINT('Ctrl Pts',(-1.18485631346681,6.00000000006835,66.5781555766083));
#8093=CARTESIAN_POINT('Ctrl Pts',(-0.992844141885393,6.00000000001632,66.5621208184677));
#8094=CARTESIAN_POINT('Ctrl Pts',(-0.923392355514658,5.99999999999751,66.5563209642829));
#8095=CARTESIAN_POINT('Ctrl Pts',(-0.853799205652419,6.00000000000023,66.5511263631302));
#8096=CARTESIAN_POINT('Ctrl Pts',(-0.784105240804896,6.00000000000023,66.5465412829041));
#8097=CARTESIAN_POINT('Ctrl Pts',(-0.557169468556095,6.00000000000023,66.5316114575713));
#8098=CARTESIAN_POINT('Ctrl Pts',(-0.328878073721691,6.00000000002498,66.5231044417488));
#8099=CARTESIAN_POINT('Ctrl Pts',(-0.100972736629075,6.0000000000241,66.521128825034));
#8100=CARTESIAN_POINT('Ctrl Pts',(-0.0701670299566568,6.00000000002398,
66.520861783157));
#8101=CARTESIAN_POINT('Ctrl Pts',(-0.0393683869893167,6.00000000002292,
66.52071399686));
#8102=CARTESIAN_POINT('Ctrl Pts',(-0.00858111222863268,6.0000000000209,
66.5206856616905));
#8103=CARTESIAN_POINT('Ctrl Pts',(-0.00379835720684805,6.00000000002059,
66.5206812598662));
#8104=CARTESIAN_POINT('Ctrl Pts',(0.000984123469690708,6.00000000002025,
66.5206797407381));
#8105=CARTESIAN_POINT('Ctrl Pts',(0.00576633055906461,6.0000000000199,66.5206811037694));
#8106=CARTESIAN_POINT('Ctrl Pts',(0.234106652522432,6.00000000000284,66.5207461856436));
#8107=CARTESIAN_POINT('Ctrl Pts',(0.461569701198186,6.00000000000127,66.5273927740508));
#8108=CARTESIAN_POINT('Ctrl Pts',(0.688691383104901,6.00000000000606,66.540566912047));
#8109=CARTESIAN_POINT('Ctrl Pts',(0.783642201262397,6.00000000000806,66.5460745111928));
#8110=CARTESIAN_POINT('Ctrl Pts',(0.8785332758493,6.00000000001171,66.5527235909363));
#8111=CARTESIAN_POINT('Ctrl Pts',(0.97340352404493,6.00000000002363,66.5605128893986));
#8112=CARTESIAN_POINT('Ctrl Pts',(1.17496698405461,6.00000000004895,66.5770622078518));
#8113=CARTESIAN_POINT('Ctrl Pts',(1.37643687431007,6.00000000008962,66.5987564371885));
#8114=CARTESIAN_POINT('Ctrl Pts',(1.57748427575531,6.00000000038885,66.625614231632));
#8115=CARTESIAN_POINT('Ctrl Pts',(1.70189213807276,6.00000000057401,66.6422337988051));
#8116=CARTESIAN_POINT('Ctrl Pts',(1.82623013085954,6.00000000051554,66.6608311538313));
#8117=CARTESIAN_POINT('Ctrl Pts',(1.95020071616002,6.00000000038028,66.6813903002302));
#8118=CARTESIAN_POINT('Ctrl Pts',(2.08632406742112,6.00000000023175,66.7039648480563));
#8119=CARTESIAN_POINT('Ctrl Pts',(2.22200401493324,6.00000000007876,66.728905060495));
#8120=CARTESIAN_POINT('Ctrl Pts',(2.35681175916437,6.0000000000386,66.7560991155276));
#8121=CARTESIAN_POINT('Ctrl Pts',(2.5182845660602,5.99999999999049,66.7886721729735));
#8122=CARTESIAN_POINT('Ctrl Pts',(2.67856245718989,5.99999999999813,66.8244779431868));
#8123=CARTESIAN_POINT('Ctrl Pts',(2.83763002040604,6.00000000000674,66.8634569456343));
#8124=CARTESIAN_POINT('Ctrl Pts',(2.86242940696275,6.00000000000808,66.8695339567467));
#8125=CARTESIAN_POINT('Ctrl Pts',(2.88719934806261,6.00000000001001,66.8756881967657));
#8126=CARTESIAN_POINT('Ctrl Pts',(2.91193975118787,6.000000000013,66.8819195489396));
#8127=CARTESIAN_POINT('Ctrl Pts',(2.98164995633899,6.00000000002142,66.8994774212269));
#8128=CARTESIAN_POINT('Ctrl Pts',(3.05112570223683,6.00000000003702,66.917647375163));
#8129=CARTESIAN_POINT('Ctrl Pts',(3.12039979918319,6.00000000008208,66.9364364740021));
#8130=CARTESIAN_POINT('Ctrl Pts',(3.36532889442497,6.0000000002414,67.0028681877584));
#8131=CARTESIAN_POINT('Ctrl Pts',(3.60744466828179,6.00000000026126,67.076928038554));
#8132=CARTESIAN_POINT('Ctrl Pts',(3.84690034723213,6.00000000016467,67.1585433863136));
#8133=CARTESIAN_POINT('Ctrl Pts',(4.09931403384456,6.00000000006285,67.2445753021256));
#8134=CARTESIAN_POINT('Ctrl Pts',(4.34877192834515,6.00000000000415,67.3390031462041));
#8135=CARTESIAN_POINT('Ctrl Pts',(4.59510054381638,6.00000000000216,67.441825521795));
#8136=CARTESIAN_POINT('Ctrl Pts',(4.64870191485623,6.00000000000173,67.4641997810532));
#8137=CARTESIAN_POINT('Ctrl Pts',(4.70214519753807,6.00000000000142,67.4869664961653));
#8138=CARTESIAN_POINT('Ctrl Pts',(4.75543960720073,6.00000000000118,67.51012947957));
#8139=CARTESIAN_POINT('Ctrl Pts',(4.92114531381994,6.00000000000044,67.5821490132658));
#8140=CARTESIAN_POINT('Ctrl Pts',(5.08541305952541,6.00000000000035,67.6579958213788));
#8141=CARTESIAN_POINT('Ctrl Pts',(5.24831190515484,6.00000000000029,67.7377664886393));
#8142=CARTESIAN_POINT('Ctrl Pts',(5.37886967950357,6.00000000000024,67.8016999114673));
#8143=CARTESIAN_POINT('Ctrl Pts',(5.50854794803044,6.00000000000024,67.8681547506109));
#8144=CARTESIAN_POINT('Ctrl Pts',(5.63737298287251,6.00000000000024,67.9372030795001));
#8145=CARTESIAN_POINT('Ctrl Pts',(5.75906631496535,6.00000000000024,68.0024289203335));
#8146=CARTESIAN_POINT('Ctrl Pts',(5.87999873423005,6.00000000000024,68.0699695887378));
#8147=CARTESIAN_POINT('Ctrl Pts',(5.9999748090223,6.00000000000024,68.139722189381));
#8148=CARTESIAN_POINT('',(6.,6.00000000000006,16.9705627484771));
#8149=CARTESIAN_POINT('',(6.,6.00000000000024,68.1396788547224));
#8150=CARTESIAN_POINT('',(8.,6.00000000000005,14.8323969741913));
#8151=CARTESIAN_POINT('Ctrl Pts',(6.,6.00000000000006,16.9705627484771));
#8152=CARTESIAN_POINT('Ctrl Pts',(6.,6.00000000000006,16.7029092618308));
#8153=CARTESIAN_POINT('Ctrl Pts',(6.06020384677459,6.00000000000006,16.3874179356908));
#8154=CARTESIAN_POINT('Ctrl Pts',(6.25585405294364,6.00000000000006,15.8960743911704));
#8155=CARTESIAN_POINT('Ctrl Pts',(6.42385919064368,6.00000000000006,15.6314481148128));
#8156=CARTESIAN_POINT('Ctrl Pts',(6.7778910457933,6.00000000000005,15.2614647616422));
#8157=CARTESIAN_POINT('Ctrl Pts',(7.02372732242562,6.00000000000005,15.0877073947429));
#8158=CARTESIAN_POINT('Ctrl Pts',(7.47536381734142,6.00000000000005,14.8921163084765));
#8159=CARTESIAN_POINT('Ctrl Pts',(7.75869936772315,6.00000000000005,14.8323969741913));
#8160=CARTESIAN_POINT('Ctrl Pts',(8.,6.00000000000005,14.8323969741913));
#8161=CARTESIAN_POINT('',(-8.,6.00000000000005,14.8323969741913));
#8162=CARTESIAN_POINT('',(8.,6.00000000000005,14.8323969741913));
#8163=CARTESIAN_POINT('Ctrl Pts',(-8.,6.00000000000005,14.8323969741913));
#8164=CARTESIAN_POINT('Ctrl Pts',(-7.75869936772315,6.00000000000005,14.8323969741913));
#8165=CARTESIAN_POINT('Ctrl Pts',(-7.47536381734142,6.00000000000005,14.8921163084765));
#8166=CARTESIAN_POINT('Ctrl Pts',(-7.02372732242562,6.00000000000005,15.0877073947429));
#8167=CARTESIAN_POINT('Ctrl Pts',(-6.7778910457933,6.00000000000005,15.2614647616422));
#8168=CARTESIAN_POINT('Ctrl Pts',(-6.42385919064368,6.00000000000006,15.6314481148128));
#8169=CARTESIAN_POINT('Ctrl Pts',(-6.25585405294364,6.00000000000006,15.8960743911704));
#8170=CARTESIAN_POINT('Ctrl Pts',(-6.06020384677459,6.00000000000006,16.3874179356908));
#8171=CARTESIAN_POINT('Ctrl Pts',(-6.,6.00000000000006,16.7029092618308));
#8172=CARTESIAN_POINT('Ctrl Pts',(-6.,6.00000000000006,16.9705627484771));
#8173=CARTESIAN_POINT('Origin',(0.,-6.,2.09488880330588E-14));
#8174=CARTESIAN_POINT('',(6.,-5.99999999999976,68.1396788547224));
#8175=CARTESIAN_POINT('',(6.,-5.99999999999994,16.9705627484772));
#8176=CARTESIAN_POINT('',(6.,-5.99999999999976,68.1396788547224));
#8177=CARTESIAN_POINT('Ctrl Pts',(6.,-6.00000000024154,68.1396788547224));
#8178=CARTESIAN_POINT('Ctrl Pts',(5.88187316617764,-6.00000000015773,68.0710098609603));
#8179=CARTESIAN_POINT('Ctrl Pts',(5.76283444829439,-6.00000000010713,68.0045242065892));
#8180=CARTESIAN_POINT('Ctrl Pts',(5.64284459885907,-6.00000000007621,67.9401565816466));
#8181=CARTESIAN_POINT('Ctrl Pts',(5.35619790196524,-6.00000000000233,67.7863871822888));
#8182=CARTESIAN_POINT('Ctrl Pts',(5.06412377906966,-5.99999999998375,67.6447057808939));
#8183=CARTESIAN_POINT('Ctrl Pts',(4.76688742341354,-6.00000000007952,67.5151296844279));
#8184=CARTESIAN_POINT('Ctrl Pts',(4.70839720439327,-6.00000000009837,67.4896316788244));
#8185=CARTESIAN_POINT('Ctrl Pts',(4.64970707509721,-6.00000000012467,67.4646024152188));
#8186=CARTESIAN_POINT('Ctrl Pts',(4.5908152128972,-6.00000000016496,67.4400433025996));
#8187=CARTESIAN_POINT('Ctrl Pts',(4.34910031027361,-6.00000000033032,67.3392432379812));
#8188=CARTESIAN_POINT('Ctrl Pts',(4.10398677156061,-6.00000000008324,67.2463175761735));
#8189=CARTESIAN_POINT('Ctrl Pts',(3.85519952238743,-6.0000000000276,67.1613594452035));
#8190=CARTESIAN_POINT('Ctrl Pts',(3.85519100898521,-6.0000000000276,67.1613565379696));
#8191=CARTESIAN_POINT('Ctrl Pts',(3.85518249557866,-6.0000000000276,67.1613536307449));
#8192=CARTESIAN_POINT('Ctrl Pts',(3.85517398216783,-6.0000000000276,67.1613507235296));
#8193=CARTESIAN_POINT('Ctrl Pts',(3.60637796813298,-5.99999999997196,67.0763902308312));
#8194=CARTESIAN_POINT('Ctrl Pts',(3.35390683475957,-5.99999999999977,66.9994050968271));
#8195=CARTESIAN_POINT('Ctrl Pts',(3.10045926892741,-5.99999999999977,66.9310858798008));
#8196=CARTESIAN_POINT('Ctrl Pts',(3.03765054448378,-5.99999999999977,66.9141551870071));
#8197=CARTESIAN_POINT('Ctrl Pts',(2.97474929840994,-5.99999999999977,66.8977478662036));
#8198=CARTESIAN_POINT('Ctrl Pts',(2.9117977058822,-5.99999999999977,66.8818763978451));
#8199=CARTESIAN_POINT('Ctrl Pts',(2.6451072621979,-5.99999999999977,66.8146379250998));
#8200=CARTESIAN_POINT('Ctrl Pts',(2.37751303071259,-5.99999999999977,66.7570207931097));
#8201=CARTESIAN_POINT('Ctrl Pts',(2.1087222951943,-5.99999999999977,66.7087297576867));
#8202=CARTESIAN_POINT('Ctrl Pts',(2.05784880463699,-5.99999999999977,66.6995898089832));
#8203=CARTESIAN_POINT('Ctrl Pts',(2.00693246700169,-5.99999999999977,66.6907837938054));
#8204=CARTESIAN_POINT('Ctrl Pts',(1.95597132257835,-5.99999999999977,66.682309504294));
#8205=CARTESIAN_POINT('Ctrl Pts',(1.82681153224339,-5.99999999999977,66.6608316220973));
#8206=CARTESIAN_POINT('Ctrl Pts',(1.69736390198919,-5.99999999999977,66.6414847915479));
#8207=CARTESIAN_POINT('Ctrl Pts',(1.56767188528546,-5.99999999999977,66.6242743320315));
#8208=CARTESIAN_POINT('Ctrl Pts',(1.37574506873217,-5.99999999999977,66.5988051567472));
#8209=CARTESIAN_POINT('Ctrl Pts',(1.1831562426598,-5.99999999999976,66.5779992309698));
#8210=CARTESIAN_POINT('Ctrl Pts',(0.989984156733664,-6.00000000000307,66.561877611386));
#8211=CARTESIAN_POINT('Ctrl Pts',(0.666428323474948,-6.00000000000862,66.5348745170574));
#8212=CARTESIAN_POINT('Ctrl Pts',(0.34123645744333,-6.00000000001651,66.5210135615664));
#8213=CARTESIAN_POINT('Ctrl Pts',(0.0138227741859248,-6.00000000000467,
66.520685928579));
#8214=CARTESIAN_POINT('Ctrl Pts',(0.0121440744646398,-6.00000000000462,
66.5206842487548));
#8215=CARTESIAN_POINT('Ctrl Pts',(0.0104653163290937,-6.00000000000456,
66.5206829246754));
#8216=CARTESIAN_POINT('Ctrl Pts',(0.00878650039514419,-6.0000000000045,
66.5206819563299));
#8217=CARTESIAN_POINT('Ctrl Pts',(-0.253515514778501,-5.99999999999504,
66.5205306598399));
#8218=CARTESIAN_POINT('Ctrl Pts',(-0.517155929846906,-5.99999999999977,
66.5290771486489));
#8219=CARTESIAN_POINT('Ctrl Pts',(-0.779619496371868,-5.99999999999977,
66.5462435242154));
#8220=CARTESIAN_POINT('Ctrl Pts',(-0.843154223039775,-5.99999999999977,
66.5503989999408));
#8221=CARTESIAN_POINT('Ctrl Pts',(-0.906642860018819,-5.99999999999672,
66.5550642741598));
#8222=CARTESIAN_POINT('Ctrl Pts',(-0.970048401227494,-6.00000000001686,
66.5602369336203));
#8223=CARTESIAN_POINT('Ctrl Pts',(-1.16857275813673,-6.00000000007993,66.5764326615223));
#8224=CARTESIAN_POINT('Ctrl Pts',(-1.36628126414112,-6.00000000065265,66.5976041035957));
#8225=CARTESIAN_POINT('Ctrl Pts',(-1.56326721620696,-6.00000000036765,66.6236701056625));
#8226=CARTESIAN_POINT('Ctrl Pts',(-1.69082862701755,-6.0000000001831,66.640549563121));
#8227=CARTESIAN_POINT('Ctrl Pts',(-1.81800947701284,-6.00000000008209,66.6594883967265));
#8228=CARTESIAN_POINT('Ctrl Pts',(-1.9449607332334,-6.00000000004002,66.6804955904311));
#8229=CARTESIAN_POINT('Ctrl Pts',(-2.07666646789127,-5.99999999999637,66.7022895290052));
#8230=CARTESIAN_POINT('Ctrl Pts',(-2.20812514567989,-5.9999999999997,66.726309580931));
#8231=CARTESIAN_POINT('Ctrl Pts',(-2.33930748785715,-6.00000000000362,66.7525690041408));
#8232=CARTESIAN_POINT('Ctrl Pts',(-2.51361784999643,-6.00000000000884,66.7874615780445));
#8233=CARTESIAN_POINT('Ctrl Pts',(-2.68751489304227,-6.00000000005027,66.8263240896056));
#8234=CARTESIAN_POINT('Ctrl Pts',(-2.86039613598336,-6.00000000005924,66.8690635323667));
#8235=CARTESIAN_POINT('Ctrl Pts',(-2.87627884399349,-6.00000000006006,66.8729900317274));
#8236=CARTESIAN_POINT('Ctrl Pts',(-2.89215298635632,-6.00000000006047,66.8769492176875));
#8237=CARTESIAN_POINT('Ctrl Pts',(-2.90801810128637,-6.00000000006037,66.8809409966382));
#8238=CARTESIAN_POINT('Ctrl Pts',(-2.97469708400514,-6.00000000005998,66.8977179163669));
#8239=CARTESIAN_POINT('Ctrl Pts',(-3.04121657240003,-6.00000000004897,66.9150706470321));
#8240=CARTESIAN_POINT('Ctrl Pts',(-3.10753849583247,-6.00000000003208,66.9329830086901));
#8241=CARTESIAN_POINT('Ctrl Pts',(-3.28869151080579,-5.99999999998595,66.9819091880242));
#8242=CARTESIAN_POINT('Ctrl Pts',(-3.46839021870641,-5.9999999999722,67.0350304856278));
#8243=CARTESIAN_POINT('Ctrl Pts',(-3.64644665283845,-6.0000000000327,67.0922158714817));
#8244=CARTESIAN_POINT('Ctrl Pts',(-3.71447004547011,-6.00000000005581,67.1140625628057));
#8245=CARTESIAN_POINT('Ctrl Pts',(-3.78225355303331,-6.00000000009765,67.1365029097764));
#8246=CARTESIAN_POINT('Ctrl Pts',(-3.84978580544277,-6.00000000021853,67.1595314065013));
#8247=CARTESIAN_POINT('Ctrl Pts',(-3.85320864030556,-6.00000000022466,67.1606985931213));
#8248=CARTESIAN_POINT('Ctrl Pts',(-3.85663082958527,-6.000000000231,67.1618672908473));
#8249=CARTESIAN_POINT('Ctrl Pts',(-3.86005237553686,-6.00000000023757,67.1630375006439));
#8250=CARTESIAN_POINT('Ctrl Pts',(-4.10768501554717,-6.00000000071298,67.2477308367549));
#8251=CARTESIAN_POINT('Ctrl Pts',(-4.35191715526809,-6.00000000647157,67.3403748233525));
#8252=CARTESIAN_POINT('Ctrl Pts',(-4.59293426136656,-6.00000000770409,67.4409174182992));
#8253=CARTESIAN_POINT('Ctrl Pts',(-4.87724480016224,-6.00000000915801,67.5595202834814));
#8254=CARTESIAN_POINT('Ctrl Pts',(-5.15698013686088,-6.00000000332805,67.6891171054417));
#8255=CARTESIAN_POINT('Ctrl Pts',(-5.43224533975829,-6.0000000013192,67.8298568940711));
#8256=CARTESIAN_POINT('Ctrl Pts',(-5.50008164654291,-6.00000000082414,67.8645407821099));
#8257=CARTESIAN_POINT('Ctrl Pts',(-5.56764646050735,-6.00000000049553,67.8999011651933));
#8258=CARTESIAN_POINT('Ctrl Pts',(-5.63494133399271,-6.00000000030077,67.9359397796821));
#8259=CARTESIAN_POINT('Ctrl Pts',(-5.75755164084124,-5.99999999994593,68.0016016251097));
#8260=CARTESIAN_POINT('Ctrl Pts',(-5.8792658872803,-5.99999999999976,68.0695150849564));
#8261=CARTESIAN_POINT('Ctrl Pts',(-5.99999401150366,-5.99999999999976,68.1396891563318));
#8262=CARTESIAN_POINT('',(-8.,-5.99999999999995,14.8323969741913));
#8263=CARTESIAN_POINT('Ctrl Pts',(-6.,-5.99999999999994,16.9705627484772));
#8264=CARTESIAN_POINT('Ctrl Pts',(-6.,-5.99999999999994,16.7029092618309));
#8265=CARTESIAN_POINT('Ctrl Pts',(-6.06020384677459,-5.99999999999994,16.3874179356908));
#8266=CARTESIAN_POINT('Ctrl Pts',(-6.25585405294364,-5.99999999999994,15.8960743911704));
#8267=CARTESIAN_POINT('Ctrl Pts',(-6.42385919064368,-5.99999999999994,15.6314481148128));
#8268=CARTESIAN_POINT('Ctrl Pts',(-6.7778910457933,-5.99999999999995,15.2614647616422));
#8269=CARTESIAN_POINT('Ctrl Pts',(-7.02372732242562,-5.99999999999995,15.0877073947429));
#8270=CARTESIAN_POINT('Ctrl Pts',(-7.47536381734142,-5.99999999999995,14.8921163084765));
#8271=CARTESIAN_POINT('Ctrl Pts',(-7.75869936772315,-5.99999999999995,14.8323969741913));
#8272=CARTESIAN_POINT('Ctrl Pts',(-8.,-5.99999999999995,14.8323969741913));
#8273=CARTESIAN_POINT('',(8.,-5.99999999999995,14.8323969741913));
#8274=CARTESIAN_POINT('',(8.,-5.99999999999995,14.8323969741913));
#8275=CARTESIAN_POINT('Ctrl Pts',(8.,-5.99999999999995,14.8323969741913));
#8276=CARTESIAN_POINT('Ctrl Pts',(7.75869936772315,-5.99999999999995,14.8323969741913));
#8277=CARTESIAN_POINT('Ctrl Pts',(7.47536381734142,-5.99999999999995,14.8921163084765));
#8278=CARTESIAN_POINT('Ctrl Pts',(7.02372732242562,-5.99999999999995,15.0877073947429));
#8279=CARTESIAN_POINT('Ctrl Pts',(6.7778910457933,-5.99999999999995,15.2614647616422));
#8280=CARTESIAN_POINT('Ctrl Pts',(6.42385919064368,-5.99999999999994,15.6314481148128));
#8281=CARTESIAN_POINT('Ctrl Pts',(6.25585405294365,-5.99999999999994,15.8960743911704));
#8282=CARTESIAN_POINT('Ctrl Pts',(6.06020384677459,-5.99999999999994,16.3874179356908));
#8283=CARTESIAN_POINT('Ctrl Pts',(6.,-5.99999999999994,16.7029092618309));
#8284=CARTESIAN_POINT('Ctrl Pts',(6.,-5.99999999999994,16.9705627484772));
#8285=CARTESIAN_POINT('Origin',(0.,0.,0.));
#8286=CARTESIAN_POINT('Origin',(0.,-9.67470971326409E-15,-79.));
#8287=CARTESIAN_POINT('',(-5.49536666714402E-12,8.23880597151339,-68.5063651759543));
#8288=CARTESIAN_POINT('Ctrl Pts',(-5.99999895840801,8.18443806084714,-70.5266960994107));
#8289=CARTESIAN_POINT('Ctrl Pts',(-5.5690974342769,8.19291945646374,-70.200366972074));
#8290=CARTESIAN_POINT('Ctrl Pts',(-4.888010383118,8.20441278535078,-69.7661879460741));
#8291=CARTESIAN_POINT('Ctrl Pts',(-3.91204062649165,8.21698677095021,-69.2997698993554));
#8292=CARTESIAN_POINT('Ctrl Pts',(-3.16398253652809,8.22477080505801,-69.0142043719821));
#8293=CARTESIAN_POINT('Ctrl Pts',(-2.39663090139138,8.23094125189423,-68.7898200788163));
#8294=CARTESIAN_POINT('Ctrl Pts',(-1.61154890932236,8.23544005858267,-68.6273289139882));
#8295=CARTESIAN_POINT('Ctrl Pts',(-0.805544548123699,8.23819902126916,-68.5281353971799));
#8296=CARTESIAN_POINT('Ctrl Pts',(-0.268787035330602,8.23880659200157,-68.5063433790642));
#8297=CARTESIAN_POINT('Ctrl Pts',(-3.18401114664506E-12,8.23880597151339,
-68.5063651759543));
#8298=CARTESIAN_POINT('',(-2.73500395030388E-10,68.5063670000441,-8.2388058234896));
#8299=CARTESIAN_POINT('Origin',(1.22464679914735E-15,0.,0.));
#8300=CARTESIAN_POINT('',(-5.99999715845766,70.5267006388891,-8.18443795663603));
#8301=CARTESIAN_POINT('Ctrl Pts',(-2.73511885838946E-10,68.5063670000441,
-8.23880582348961));
#8302=CARTESIAN_POINT('Ctrl Pts',(-0.00373884108269842,68.5063664082688,
-8.2388058387049));
#8303=CARTESIAN_POINT('Ctrl Pts',(-0.00747734760339464,68.5063679389705,
-8.23880579472993));
#8304=CARTESIAN_POINT('Ctrl Pts',(-0.0112155109279515,68.5063715920789,
-8.23880569156401));
#8305=CARTESIAN_POINT('Ctrl Pts',(-0.0121232949516723,68.506372479208,-8.23880566651096));
#8306=CARTESIAN_POINT('Ctrl Pts',(-0.0130310587363146,68.5063734915004,
-8.23880563796729));
#8307=CARTESIAN_POINT('Ctrl Pts',(-0.0139388023081085,68.506374628946,-8.23880560593331));
#8308=CARTESIAN_POINT('Ctrl Pts',(-0.282917995094099,68.5067116725797,-8.23879611374476));
#8309=CARTESIAN_POINT('Ctrl Pts',(-0.550108573868126,68.518036776789,-8.2384805240124));
#8310=CARTESIAN_POINT('Ctrl Pts',(-0.81624500940925,68.5400862637072,-8.23786687734688));
#8311=CARTESIAN_POINT('Ctrl Pts',(-0.818721129250123,68.5402914110104,-8.23786116800956));
#8312=CARTESIAN_POINT('Ctrl Pts',(-0.821197157164274,68.5404974866639,-8.2378554328535));
#8313=CARTESIAN_POINT('Ctrl Pts',(-0.823673093694567,68.5407044904533,-8.23784967188635));
#8314=CARTESIAN_POINT('Ctrl Pts',(-1.08731389025658,68.562746511014,-8.23723623694985));
#8315=CARTESIAN_POINT('Ctrl Pts',(-1.34991844716521,68.595312828994,-8.23633012591871));
#8316=CARTESIAN_POINT('Ctrl Pts',(-1.61124780956339,68.6384063740778,-8.23513519709042));
#8317=CARTESIAN_POINT('Ctrl Pts',(-1.61706443909913,68.6393655437051,-8.23510860054477));
#8318=CARTESIAN_POINT('Ctrl Pts',(-1.6228804407311,68.6403299288959,-8.2350818604792));
#8319=CARTESIAN_POINT('Ctrl Pts',(-1.62869581330632,68.6412995298965,-8.23505497690792));
#8320=CARTESIAN_POINT('Ctrl Pts',(-1.88660702918973,68.6843012412662,-8.23386269310027));
#8321=CARTESIAN_POINT('Ctrl Pts',(-2.14328123564365,68.7375593459786,-8.2323882178511));
#8322=CARTESIAN_POINT('Ctrl Pts',(-2.39893596892781,68.8014424014476,-8.23062526198179));
#8323=CARTESIAN_POINT('Ctrl Pts',(-2.40804734805945,68.8037191546725,-8.23056243130735));
#8324=CARTESIAN_POINT('Ctrl Pts',(-2.41715726285983,68.8060093642543,-8.23049923764878));
#8325=CARTESIAN_POINT('Ctrl Pts',(-2.42626571371847,68.8083130436881,-8.23043568090945));
#8326=CARTESIAN_POINT('Ctrl Pts',(-2.67849247305856,68.8721054060963,-8.22867569881752));
#8327=CARTESIAN_POINT('Ctrl Pts',(-2.92959437693503,68.9462290809758,-8.22663723937388));
#8328=CARTESIAN_POINT('Ctrl Pts',(-3.17579288399155,69.0294813142028,-8.22436060167555));
#8329=CARTESIAN_POINT('Ctrl Pts',(-3.18802172175186,69.0336165060262,-8.22424751962081));
#8330=CARTESIAN_POINT('Ctrl Pts',(-3.2002384390651,69.0377742047295,-8.22413384470118));
#8331=CARTESIAN_POINT('Ctrl Pts',(-3.21244258772405,69.0419542652417,-8.22401958158434));
#8332=CARTESIAN_POINT('Ctrl Pts',(-3.47069841243532,69.1304098392505,-8.2216016238637));
#8333=CARTESIAN_POINT('Ctrl Pts',(-3.72332652714384,69.2288791839828,-8.21892027353038));
#8334=CARTESIAN_POINT('Ctrl Pts',(-3.97115318499118,69.3372405923039,-8.21598633637045));
#8335=CARTESIAN_POINT('Ctrl Pts',(-4.20020274943883,69.4373917769846,-8.21327469495772));
#8336=CARTESIAN_POINT('Ctrl Pts',(-4.42515017140143,69.545992763761,-8.21034729396852));
#8337=CARTESIAN_POINT('Ctrl Pts',(-4.64577000290152,69.6628850216051,-8.20721520875059));
#8338=CARTESIAN_POINT('Ctrl Pts',(-4.66424094621694,69.6726715863666,-8.20695298133374));
#8339=CARTESIAN_POINT('Ctrl Pts',(-4.68267694908691,69.6825138207613,-8.20668942620729));
#8340=CARTESIAN_POINT('Ctrl Pts',(-4.7010785817278,69.6924119031607,-8.20642454061931));
#8341=CARTESIAN_POINT('Ctrl Pts',(-4.83443960450597,69.764145668207,-8.2045048515558));
#8342=CARTESIAN_POINT('Ctrl Pts',(-4.96599736269102,69.83880901757,-8.20251537469265));
#8343=CARTESIAN_POINT('Ctrl Pts',(-5.09608337284685,69.9166283180189,-8.20045120283686));
#8344=CARTESIAN_POINT('Ctrl Pts',(-5.19900771676893,69.9781991236234,-8.19881802542029));
#8345=CARTESIAN_POINT('Ctrl Pts',(-5.30101022676462,70.0417463620704,-8.19713806766012));
#8346=CARTESIAN_POINT('Ctrl Pts',(-5.40224525221829,70.1074031078172,-8.19540839604894));
#8347=CARTESIAN_POINT('Ctrl Pts',(-5.52569971532715,70.1874704388553,-8.1932990897179));
#8348=CARTESIAN_POINT('Ctrl Pts',(-5.64801488356454,70.2706747960204,-8.19111584759849));
#8349=CARTESIAN_POINT('Ctrl Pts',(-5.76875558037752,70.356772821631,-8.18886619176866));
#8350=CARTESIAN_POINT('Ctrl Pts',(-5.84653233268286,70.4122340289011,-8.1874170455498));
#8351=CARTESIAN_POINT('Ctrl Pts',(-5.92365514224985,70.4688966414595,-8.18594032623917));
#8352=CARTESIAN_POINT('Ctrl Pts',(-5.99999716495239,70.5267006438067,-8.18443795650821));
#8353=CARTESIAN_POINT('',(-6.,70.5266968882281,8.18443804032995));
#8354=CARTESIAN_POINT('Origin',(-6.,-3.53369596958238E-16,0.));
#8355=CARTESIAN_POINT('',(-8.95159733014031E-12,68.5063647597673,8.23880598322944));
#8356=CARTESIAN_POINT('Ctrl Pts',(-5.99999948661478,70.5266964994307,8.18443805045074));
#8357=CARTESIAN_POINT('Ctrl Pts',(-5.78451154162507,70.3635037543157,8.18867948064694));
#8358=CARTESIAN_POINT('Ctrl Pts',(-5.34212806448152,70.055768219971,8.19674757400964));
#8359=CARTESIAN_POINT('Ctrl Pts',(-4.64059859463673,69.6477395339077,8.2076055215689));
#8360=CARTESIAN_POINT('Ctrl Pts',(-3.91292633842418,69.3002864631745,8.21697301436391));
#8361=CARTESIAN_POINT('Ctrl Pts',(-3.16585416162398,69.0148381621378,8.22475339508119));
#8362=CARTESIAN_POINT('Ctrl Pts',(-2.39835642218803,68.7901683634025,8.23093161161829));
#8363=CARTESIAN_POINT('Ctrl Pts',(-1.6087834219025,68.6267990516475,8.23545474346867));
#8364=CARTESIAN_POINT('Ctrl Pts',(-0.804180861593639,68.5281198274787,8.23819947080704));
#8365=CARTESIAN_POINT('Ctrl Pts',(-0.268573138561608,68.5063141973659,8.23880740764904));
#8366=CARTESIAN_POINT('Ctrl Pts',(-8.95159733014031E-12,68.5063647597673,
8.23880598322944));
#8367=CARTESIAN_POINT('',(-2.38940561989992E-10,8.23880549026604,68.5063639612443));
#8368=CARTESIAN_POINT('Origin',(1.22464679914735E-15,0.,0.));
#8369=CARTESIAN_POINT('Ctrl Pts',(-2.38940450967676E-10,8.23880549026604,
68.5063639612443));
#8370=CARTESIAN_POINT('Ctrl Pts',(-0.00119743047815034,8.23880548637175,
68.5063641815433));
#8371=CARTESIAN_POINT('Ctrl Pts',(-0.00239488142112834,8.2388054764133,
68.5063646198442));
#8372=CARTESIAN_POINT('Ctrl Pts',(-0.00359235313103486,8.23880546039038,
68.5063652761552));
#8373=CARTESIAN_POINT('Ctrl Pts',(-0.00477852616968188,8.23880544451865,
68.5063659262736));
#8374=CARTESIAN_POINT('Ctrl Pts',(-0.00596471919577684,8.23880542267338,
68.5063667903101));
#8375=CARTESIAN_POINT('Ctrl Pts',(-0.00715093227137261,8.23880539485422,
68.506367868272));
#8376=CARTESIAN_POINT('Ctrl Pts',(-0.275542599110005,8.23879910051263,68.5066117671079));
#8377=CARTESIAN_POINT('Ctrl Pts',(-0.544960513818001,8.23848697859665,68.5178073781331));
#8378=CARTESIAN_POINT('Ctrl Pts',(-0.811826492207112,8.23787592190724,68.5397251334166));
#8379=CARTESIAN_POINT('Ctrl Pts',(-0.817008824069481,8.23786405565674,68.5401507593515));
#8380=CARTESIAN_POINT('Ctrl Pts',(-0.822190223933388,8.23785207545356,68.540580431239));
#8381=CARTESIAN_POINT('Ctrl Pts',(-0.827370663690959,8.23783998143978,68.5410141473606));
#8382=CARTESIAN_POINT('Ctrl Pts',(-1.06376993820737,8.23728809468556,68.5608059374966));
#8383=CARTESIAN_POINT('Ctrl Pts',(-1.29816894019248,8.2364990940397,68.5890236262271));
#8384=CARTESIAN_POINT('Ctrl Pts',(-1.53073410795179,8.23548929589195,68.6254521884976));
#8385=CARTESIAN_POINT('Ctrl Pts',(-1.55667432227247,8.23537666346025,68.6295154139659));
#8386=CARTESIAN_POINT('Ctrl Pts',(-1.5825917325838,8.23526128548904,68.6336807394219));
#8387=CARTESIAN_POINT('Ctrl Pts',(-1.60848657744125,8.23514318567388,68.6379478275793));
#8388=CARTESIAN_POINT('Ctrl Pts',(-1.61754348689097,8.23510187940857,68.6394402725531));
#8389=CARTESIAN_POINT('Ctrl Pts',(-1.62659786881208,8.23506022841665,68.6409452057524));
#8390=CARTESIAN_POINT('Ctrl Pts',(-1.63564974610698,8.23501823312477,68.6424626167318));
#8391=CARTESIAN_POINT('Ctrl Pts',(-1.90269718744703,8.23377929286099,68.6872291006701));
#8392=CARTESIAN_POINT('Ctrl Pts',(-2.16756507620287,8.23224073153665,68.7428541162553));
#8393=CARTESIAN_POINT('Ctrl Pts',(-2.43002969761608,8.23040991820687,68.8092649879185));
#8394=CARTESIAN_POINT('Ctrl Pts',(-2.67563111594158,8.2286967335953,68.8714089987376));
#8395=CARTESIAN_POINT('Ctrl Pts',(-2.91912792037934,8.22672764247879,68.9429974373362));
#8396=CARTESIAN_POINT('Ctrl Pts',(-3.16108135489304,8.22449604172108,69.0244973202163));
#8397=CARTESIAN_POINT('Ctrl Pts',(-3.17757512971591,8.2243439152573,69.0300531029602));
#8398=CARTESIAN_POINT('Ctrl Pts',(-3.19405954559071,8.22419061910876,69.0356542108646));
#8399=CARTESIAN_POINT('Ctrl Pts',(-3.21053495270791,8.22403614735284,69.0413008166669));
#8400=CARTESIAN_POINT('Ctrl Pts',(-3.38604792150681,8.22239055545433,69.1014542648307));
#8401=CARTESIAN_POINT('Ctrl Pts',(-3.56053902191876,8.2206116630597,69.166766732304));
#8402=CARTESIAN_POINT('Ctrl Pts',(-3.7329361227573,8.21870979242949,69.2368236563124));
#8403=CARTESIAN_POINT('Ctrl Pts',(-3.79419891986031,8.21803394629305,69.2617189886603));
#8404=CARTESIAN_POINT('Ctrl Pts',(-3.85519719392959,8.21734255808504,69.2872139255654));
#8405=CARTESIAN_POINT('Ctrl Pts',(-3.9158822437057,8.21663605348593,69.3132913313463));
#8406=CARTESIAN_POINT('Ctrl Pts',(-3.93571269242953,8.21640518437932,69.3218128149752));
#8407=CARTESIAN_POINT('Ctrl Pts',(-3.95551155625911,8.21617269798135,69.3303973027179));
#8408=CARTESIAN_POINT('Ctrl Pts',(-3.97527663721697,8.21593862172726,69.3390440387009));
#8409=CARTESIAN_POINT('Ctrl Pts',(-4.18546974883883,8.21344932171843,69.4309983466808));
#8410=CARTESIAN_POINT('Ctrl Pts',(-4.39183988326306,8.21078011928237,69.5299962380484));
#8411=CARTESIAN_POINT('Ctrl Pts',(-4.59434450063668,8.20794530577172,69.6358149303183));
#8412=CARTESIAN_POINT('Ctrl Pts',(-4.61044583130454,8.20771990711015,69.6442286730624));
#8413=CARTESIAN_POINT('Ctrl Pts',(-4.62652273854098,8.20749346207156,69.6526855137308));
#8414=CARTESIAN_POINT('Ctrl Pts',(-4.6425752083125,8.20726597815253,69.6611853284648));
#8415=CARTESIAN_POINT('Ctrl Pts',(-4.6646451753276,8.20695321864193,69.6728714199812));
#8416=CARTESIAN_POINT('Ctrl Pts',(-4.68666871769243,8.20663846427466,69.6846386242432));
#8417=CARTESIAN_POINT('Ctrl Pts',(-4.70864603612887,8.20632172869146,69.6964867360917));
#8418=CARTESIAN_POINT('Ctrl Pts',(-5.02435114272387,8.20177180867526,69.8666853626846));
#8419=CARTESIAN_POINT('Ctrl Pts',(-5.33051997376249,8.19681310827977,70.0535759591058));
#8420=CARTESIAN_POINT('Ctrl Pts',(-5.62708060760958,8.19146556534272,70.2574709713756));
#8421=CARTESIAN_POINT('Ctrl Pts',(-5.75312566204789,8.18919273724726,70.3441310165336));
#8422=CARTESIAN_POINT('Ctrl Pts',(-5.87743471628307,8.18684965924949,70.4338633607541));
#8423=CARTESIAN_POINT('Ctrl Pts',(-6.00000075752689,8.18443783045391,70.5266944330751));
#8424=CARTESIAN_POINT('',(4.16525128190542E-10,-8.23880590935122,68.5063673993547));
#8425=CARTESIAN_POINT('Ctrl Pts',(-5.99999999999998,-8.18443804034557,70.5266968882263));
#8426=CARTESIAN_POINT('Ctrl Pts',(-5.78418052149934,-8.18868599659508,70.3632530453486));
#8427=CARTESIAN_POINT('Ctrl Pts',(-5.33854958945116,-8.19680831145233,70.0534670788763));
#8428=CARTESIAN_POINT('Ctrl Pts',(-4.41053460175808,-8.21115661661037,69.5143250649606));
#8429=CARTESIAN_POINT('Ctrl Pts',(-3.43120662489604,-8.22261256046406,69.0927024818813));
#8430=CARTESIAN_POINT('Ctrl Pts',(-2.39407107542595,-8.23096914645052,68.7888010655747));
#8431=CARTESIAN_POINT('Ctrl Pts',(-1.60026509897427,-8.23549084886545,68.6255002091326));
#8432=CARTESIAN_POINT('Ctrl Pts',(-0.80294392845351,-8.23820151213957,68.5280473459781));
#8433=CARTESIAN_POINT('Ctrl Pts',(-0.265147204082705,-8.23880460260968,
68.5064140674028));
#8434=CARTESIAN_POINT('Ctrl Pts',(4.16541472538293E-10,-8.23880590935122,
68.5063673993548));
#8435=CARTESIAN_POINT('',(-3.51061826131195E-10,-68.5063672600388,8.23880581768755));
#8436=CARTESIAN_POINT('Origin',(1.22464679914735E-15,0.,0.));
#8437=CARTESIAN_POINT('Ctrl Pts',(-3.51073400206478E-10,-68.5063672600388,
8.23880581768755));
#8438=CARTESIAN_POINT('Ctrl Pts',(-0.00385818621438253,-68.5063665769295,
8.23880583540891));
#8439=CARTESIAN_POINT('Ctrl Pts',(-0.00771604492353719,-68.5063681582155,
8.23880578998357));
#8440=CARTESIAN_POINT('Ctrl Pts',(-0.0115735656074801,-68.5063720042282,
8.23880568139922));
#8441=CARTESIAN_POINT('Ctrl Pts',(-0.0116031125215163,-68.506372033687,
8.23880568056751));
#8442=CARTESIAN_POINT('Ctrl Pts',(-0.0116326594157389,-68.5063720632786,
8.2388056797321));
#8443=CARTESIAN_POINT('Ctrl Pts',(-0.0116622062901124,-68.5063720930031,
8.23880567889298));
#8444=CARTESIAN_POINT('Ctrl Pts',(-0.28104379280587,-68.5066430940673,8.23879802856396));
#8445=CARTESIAN_POINT('Ctrl Pts',(-0.548776288907163,-68.5179577377854,
8.23848251126927));
#8446=CARTESIAN_POINT('Ctrl Pts',(-0.815115448555507,-68.5399926087912,
8.23786943479957));
#8447=CARTESIAN_POINT('Ctrl Pts',(-0.818638638156674,-68.5402840906314,
8.23786132489698));
#8448=CARTESIAN_POINT('Ctrl Pts',(-0.822161582922775,-68.540577448376,8.23785316286225));
#8449=CARTESIAN_POINT('Ctrl Pts',(-0.825684283357457,-68.5408726812731,
8.23784494871921));
#8450=CARTESIAN_POINT('Ctrl Pts',(-1.08846376352508,-68.5628958844056,8.23723220622846));
#8451=CARTESIAN_POINT('Ctrl Pts',(-1.34988356665061,-68.5953539573717,8.23632949102674));
#8452=CARTESIAN_POINT('Ctrl Pts',(-1.60969559173261,-68.6381510212431,8.2351425283051));
#8453=CARTESIAN_POINT('Ctrl Pts',(-1.61671526827113,-68.6393073247093,8.23511045860252));
#8454=CARTESIAN_POINT('Ctrl Pts',(-1.62373379075566,-68.6404711784755,8.2350781807139));
#8455=CARTESIAN_POINT('Ctrl Pts',(-1.63075115562209,-68.6416425809445,8.23504569477409));
#8456=CARTESIAN_POINT('Ctrl Pts',(-1.88694202943979,-68.6844082954009,8.23385969383694));
#8457=CARTESIAN_POINT('Ctrl Pts',(-2.14159007557437,-68.7372339187662,8.2323964294449));
#8458=CARTESIAN_POINT('Ctrl Pts',(-2.39544154112822,-68.8005695892671,8.23064983883997));
#8459=CARTESIAN_POINT('Ctrl Pts',(-2.40589777583131,-68.8031784086978,8.2305778961342));
#8460=CARTESIAN_POINT('Ctrl Pts',(-2.41635237751087,-68.8058049920654,8.23050547446862));
#8461=CARTESIAN_POINT('Ctrl Pts',(-2.42680539922861,-68.8084493687539,8.23043257324636));
#8462=CARTESIAN_POINT('Ctrl Pts',(-2.67707698890509,-68.8717623872676,8.22868713491521));
#8463=CARTESIAN_POINT('Ctrl Pts',(-2.92644200671099,-68.9452735301382,8.22666684341862));
#8464=CARTESIAN_POINT('Ctrl Pts',(-3.17155833115999,-69.0280482116615,8.22440186183105));
#8465=CARTESIAN_POINT('Ctrl Pts',(-3.18529986316834,-69.0326886652836,8.22427488409078));
#8466=CARTESIAN_POINT('Ctrl Pts',(-3.19902855252207,-69.0373584099793,8.22414713390775));
#8467=CARTESIAN_POINT('Ctrl Pts',(-3.21274375596388,-69.0420572713038,8.22401861745451));
#8468=CARTESIAN_POINT('Ctrl Pts',(-3.43326552071907,-69.1176085524791,8.22195224817393));
#8469=CARTESIAN_POINT('Ctrl Pts',(-3.65029895515285,-69.2006910611612,8.21968767912429));
#8470=CARTESIAN_POINT('Ctrl Pts',(-3.86355207639196,-69.2909505112194,8.21724088229277));
#8471=CARTESIAN_POINT('Ctrl Pts',(-3.88349996596054,-69.2993934616991,8.21701200670723));
#8472=CARTESIAN_POINT('Ctrl Pts',(-3.90341479510208,-69.3078991761863,8.21678153750259));
#8473=CARTESIAN_POINT('Ctrl Pts',(-3.92329633543422,-69.316467344228,8.21654948826908));
#8474=CARTESIAN_POINT('Ctrl Pts',(-3.93993217901766,-69.3236367436286,8.21635532148483));
#8475=CARTESIAN_POINT('Ctrl Pts',(-3.9565447498138,-69.3308498856566,8.21616003519082));
#8476=CARTESIAN_POINT('Ctrl Pts',(-3.97313405731919,-69.338106650427,8.2159636358534));
#8477=CARTESIAN_POINT('Ctrl Pts',(-4.20150197396974,-69.4380030597072,8.21326000838113));
#8478=CARTESIAN_POINT('Ctrl Pts',(-4.42546345991262,-69.546162167036,8.21034555688662));
#8479=CARTESIAN_POINT('Ctrl Pts',(-4.64518491558962,-69.6625713356289,8.20722979971519));
#8480=CARTESIAN_POINT('Ctrl Pts',(-4.66456114572406,-69.6728369277326,8.20695503534223));
#8481=CARTESIAN_POINT('Ctrl Pts',(-4.68390071403998,-69.6831647622597,8.20667874858075));
#8482=CARTESIAN_POINT('Ctrl Pts',(-4.70320400447882,-69.6935549071169,8.20640094242959));
#8483=CARTESIAN_POINT('Ctrl Pts',(-4.86547624806854,-69.7808991929293,8.20406557750431));
#8484=CARTESIAN_POINT('Ctrl Pts',(-5.02518681123594,-69.8726431417192,8.20162293160604));
#8485=CARTESIAN_POINT('Ctrl Pts',(-5.18266532395224,-69.9690359345141,8.19906977102499));
#8486=CARTESIAN_POINT('Ctrl Pts',(-5.25664466501042,-70.0143187808576,8.19787036207616));
#8487=CARTESIAN_POINT('Ctrl Pts',(-5.33013106871451,-70.0606282200054,8.1966465478237));
#8488=CARTESIAN_POINT('Ctrl Pts',(-5.40315693610489,-70.1079936559069,8.19539790722249));
#8489=CARTESIAN_POINT('Ctrl Pts',(-5.55655477109986,-70.2074892946516,8.19277501794013));
#8490=CARTESIAN_POINT('Ctrl Pts',(-5.70792279166802,-70.3116421098362,8.19004263268351));
#8491=CARTESIAN_POINT('Ctrl Pts',(-5.85676761348635,-70.4202342062778,8.18721006457127));
#8492=CARTESIAN_POINT('Ctrl Pts',(-5.90477990751254,-70.4552623355709,8.18629637411572));
#8493=CARTESIAN_POINT('Ctrl Pts',(-5.95252939627508,-70.4907526632035,8.18537225351234));
#8494=CARTESIAN_POINT('Ctrl Pts',(-5.99999865521153,-70.5266986694858,8.18443799940374));
#8495=CARTESIAN_POINT('',(-1.22464679914735E-15,-68.5063652081765,-8.2388061006397));
#8496=CARTESIAN_POINT('Ctrl Pts',(-5.99999923045746,-70.5266963054383,-8.18443805549265));
#8497=CARTESIAN_POINT('Ctrl Pts',(-5.87027903212654,-70.4284569638484,-8.18699132655943));
#8498=CARTESIAN_POINT('Ctrl Pts',(-5.73842754629939,-70.3335701958321,-8.18947252824115));
#8499=CARTESIAN_POINT('Ctrl Pts',(-5.60435418714887,-70.2419484360896,-8.19187705488044));
#8500=CARTESIAN_POINT('Ctrl Pts',(-5.51565628121315,-70.1813349161569,-8.1934677995222));
#8501=CARTESIAN_POINT('Ctrl Pts',(-5.42598523691919,-70.122151187232,-8.19502506306265));
#8502=CARTESIAN_POINT('Ctrl Pts',(-5.3353077250708,-70.0643821800456,-8.19654852892693));
#8503=CARTESIAN_POINT('Ctrl Pts',(-5.2178641440315,-69.9895609929755,-8.19852168944981));
#8504=CARTESIAN_POINT('Ctrl Pts',(-5.09872782901844,-69.9171169607333,-8.20043878610134));
#8505=CARTESIAN_POINT('Ctrl Pts',(-4.97824262075468,-69.8472641180671,-8.20229660945547));
#8506=CARTESIAN_POINT('Ctrl Pts',(-4.865086125733,-69.7816601907692,-8.20404142761325));
#8507=CARTESIAN_POINT('Ctrl Pts',(-4.75074030582435,-69.7183415425653,-8.20573394692875));
#8508=CARTESIAN_POINT('Ctrl Pts',(-4.63551013050863,-69.6574489672838,-8.20736745994599));
#8509=CARTESIAN_POINT('Ctrl Pts',(-4.46498601115885,-69.5673366963759,-8.20978482473736));
#8510=CARTESIAN_POINT('Ctrl Pts',(-4.2925273749644,-69.4825256560631,-8.21207037874011));
#8511=CARTESIAN_POINT('Ctrl Pts',(-4.11819334568071,-69.4029361694811,-8.21422081851545));
#8512=CARTESIAN_POINT('Ctrl Pts',(-3.94271063860926,-69.3228222719408,-8.21638542742584));
#8513=CARTESIAN_POINT('Ctrl Pts',(-3.76532722073528,-69.2479986650071,-8.21841309567276));
#8514=CARTESIAN_POINT('Ctrl Pts',(-3.58607414262684,-69.1784279779047,-8.22030371422339));
#8515=CARTESIAN_POINT('Ctrl Pts',(-3.44647633668207,-69.1242480699218,-8.22177608058012));
#8516=CARTESIAN_POINT('Ctrl Pts',(-3.30574393103558,-69.073254855566,-8.22316538895211));
#8517=CARTESIAN_POINT('Ctrl Pts',(-3.16388256600053,-69.0254505692774,-8.22447316069163));
#8518=CARTESIAN_POINT('Ctrl Pts',(-3.01568852837794,-68.9755123059664,-8.22583931118877));
#8519=CARTESIAN_POINT('Ctrl Pts',(-2.86626984965028,-68.9290537059868,-8.22711708905403));
#8520=CARTESIAN_POINT('Ctrl Pts',(-2.71547697134612,-68.8860638985536,-8.22829946064218));
#8521=CARTESIAN_POINT('Ctrl Pts',(-2.60934779248849,-68.855807343911,-8.2291316227918));
#8522=CARTESIAN_POINT('Ctrl Pts',(-2.50253757802254,-68.8272700577375,-8.22991663042879));
#8523=CARTESIAN_POINT('Ctrl Pts',(-2.39499130075912,-68.8004633954027,-8.23065360525647));
#8524=CARTESIAN_POINT('Ctrl Pts',(-2.26395851548226,-68.7678025565611,-8.23155152442956));
#8525=CARTESIAN_POINT('Ctrl Pts',(-2.13182992580535,-68.7377160415585,-8.23237878926188));
#8526=CARTESIAN_POINT('Ctrl Pts',(-1.9989917728853,-68.7103301969358,-8.23313611364337));
#8527=CARTESIAN_POINT('Ctrl Pts',(-1.86789016177572,-68.683302356871,-8.23388353781604));
#8528=CARTESIAN_POINT('Ctrl Pts',(-1.73609775085767,-68.6589050200765,-8.23456284263883));
#8529=CARTESIAN_POINT('Ctrl Pts',(-1.60399728261137,-68.6372115535411,-8.23516858331626));
#8530=CARTESIAN_POINT('Ctrl Pts',(-1.38764322858426,-68.6016820093,-8.23616066497192));
#8531=CARTESIAN_POINT('Ctrl Pts',(-1.17046576101213,-68.5733904177854,-8.23695222102039));
#8532=CARTESIAN_POINT('Ctrl Pts',(-0.952624108263045,-68.5523229098841,
-8.23753982863067));
#8533=CARTESIAN_POINT('Ctrl Pts',(-0.734950166798859,-68.5312716213733,
-8.23812698385535));
#8534=CARTESIAN_POINT('Ctrl Pts',(-0.516612293295068,-68.5174332298595,
-8.23851049823526));
#8535=CARTESIAN_POINT('Ctrl Pts',(-0.297763899889859,-68.5108453651861,
-8.23868919922455));
#8536=CARTESIAN_POINT('Ctrl Pts',(-0.198609217040279,-68.5078605699944,
-8.23877016413201));
#8537=CARTESIAN_POINT('Ctrl Pts',(-0.0993497327048553,-68.5063648454567,
-8.23880911668573));
#8538=CARTESIAN_POINT('Ctrl Pts',(-1.22464679914735E-15,-68.5063652081765,
-8.23880610063971));
#8539=CARTESIAN_POINT('',(-7.6571373978539E-15,-8.23880518655814,-68.5063653181071));
#8540=CARTESIAN_POINT('Origin',(1.22464679914735E-15,0.,0.));
#8541=CARTESIAN_POINT('Ctrl Pts',(-7.6571373978539E-15,-8.23880518655807,
-68.5063653181071));
#8542=CARTESIAN_POINT('Ctrl Pts',(-0.00206351045186059,-8.23880544768633,
-68.5063652867029));
#8543=CARTESIAN_POINT('Ctrl Pts',(-0.00412693915927323,-8.23880569090796,
-68.506365900766));
#8544=CARTESIAN_POINT('Ctrl Pts',(-0.0061902852373708,-8.2388059161998,
-68.5063671601456));
#8545=CARTESIAN_POINT('Ctrl Pts',(-0.168945921413918,-8.23882368709946,
-68.5064664993328));
#8546=CARTESIAN_POINT('Ctrl Pts',(-0.331181753910835,-8.23872945968339,
-68.5105766381394));
#8547=CARTESIAN_POINT('Ctrl Pts',(-0.493021483442529,-8.23851680360619,
-68.5186485086519));
#8548=CARTESIAN_POINT('Ctrl Pts',(-0.655074028978294,-8.23830386789052,
-68.5267309935124));
#8549=CARTESIAN_POINT('Ctrl Pts',(-0.816729897949388,-8.23797219477017,
-68.5387856576554));
#8550=CARTESIAN_POINT('Ctrl Pts',(-0.978113579330973,-8.23752036276245,
-68.5548152559583));
#8551=CARTESIAN_POINT('Ctrl Pts',(-1.13917076696477,-8.23706944485165,-68.5708124249375));
#8552=CARTESIAN_POINT('Ctrl Pts',(-1.29995732955209,-8.23649886288153,-68.5907685178097));
#8553=CARTESIAN_POINT('Ctrl Pts',(-1.46059033272571,-8.23581211997273,-68.614737415174));
#8554=CARTESIAN_POINT('Ctrl Pts',(-1.50766644276116,-8.23561085881157,-68.6217618897679));
#8555=CARTESIAN_POINT('Ctrl Pts',(-1.55472929520138,-8.2353996525357,-68.6291313474598));
#8556=CARTESIAN_POINT('Ctrl Pts',(-1.60178163876484,-8.23517866757182,-68.6368479678193));
#8557=CARTESIAN_POINT('Ctrl Pts',(-1.74949257113952,-8.23448493177496,-68.6610726737907));
#8558=CARTESIAN_POINT('Ctrl Pts',(-1.89710107729826,-8.23369575365773,-68.6887235288312));
#8559=CARTESIAN_POINT('Ctrl Pts',(-2.04420312931326,-8.23282291319157,-68.7197671066736));
#8560=CARTESIAN_POINT('Ctrl Pts',(-2.19121197202044,-8.23195062578946,-68.7507910141554));
#8561=CARTESIAN_POINT('Ctrl Pts',(-2.33771464560452,-8.23099476748653,-68.7852032984919));
#8562=CARTESIAN_POINT('Ctrl Pts',(-2.48331624371162,-8.22996030290718,-68.822919674804));
#8563=CARTESIAN_POINT('Ctrl Pts',(-2.62904439646648,-8.22892493918728,-68.8606688336046));
#8564=CARTESIAN_POINT('Ctrl Pts',(-2.7738695573344,-8.22781081116615,-68.901727740215));
#8565=CARTESIAN_POINT('Ctrl Pts',(-2.91740947016524,-8.22661635650124,-68.9459618822334));
#8566=CARTESIAN_POINT('Ctrl Pts',(-3.00103310871868,-8.22592048980328,-68.9717318568064));
#8567=CARTESIAN_POINT('Ctrl Pts',(-3.08422081663934,-8.2251972393183,-68.9985785790516));
#8568=CARTESIAN_POINT('Ctrl Pts',(-3.16689985036813,-8.22444532483442,-69.0264678697792));
#8569=CARTESIAN_POINT('Ctrl Pts',(-3.32589426532498,-8.22299936933555,-69.0800998640443));
#8570=CARTESIAN_POINT('Ctrl Pts',(-3.48301497421291,-8.22144690169077,-69.1375833051657));
#8571=CARTESIAN_POINT('Ctrl Pts',(-3.63837777161623,-8.21978673379442,-69.1988932866378));
#8572=CARTESIAN_POINT('Ctrl Pts',(-3.79404440644263,-8.21812331916755,-69.2603231698309));
#8573=CARTESIAN_POINT('Ctrl Pts',(-3.94794670471723,-8.21635180738967,-69.325594744792));
#8574=CARTESIAN_POINT('Ctrl Pts',(-4.10018577887777,-8.21447595386902,-69.3947327342989));
#8575=CARTESIAN_POINT('Ctrl Pts',(-4.25226186536004,-8.21260210864363,-69.4637967044356));
#8576=CARTESIAN_POINT('Ctrl Pts',(-4.40267872776132,-8.2106241749733,-69.5367190183991));
#8577=CARTESIAN_POINT('Ctrl Pts',(-4.5515151235918,-8.20855041683867,-69.6135711035785));
#8578=CARTESIAN_POINT('Ctrl Pts',(-4.58036246705801,-8.20814848280337,-69.628466509268));
#8579=CARTESIAN_POINT('Ctrl Pts',(-4.6091503609389,-8.20774296187061,-69.6435096758942));
#8580=CARTESIAN_POINT('Ctrl Pts',(-4.6378792610473,-8.20733393235838,-69.6587013169032));
#8581=CARTESIAN_POINT('Ctrl Pts',(-4.80509780639098,-8.20495314785988,-69.7471253116028));
#8582=CARTESIAN_POINT('Ctrl Pts',(-4.97030250657127,-8.20245399782115,-69.8405765183875));
#8583=CARTESIAN_POINT('Ctrl Pts',(-5.13305779370999,-8.1998458336701,-69.9388954647287));
#8584=CARTESIAN_POINT('Ctrl Pts',(-5.29568134156507,-8.19723978064971,-70.0371348286011));
#8585=CARTESIAN_POINT('Ctrl Pts',(-5.45585907554819,-8.19452484502024,-70.1402339115534));
#8586=CARTESIAN_POINT('Ctrl Pts',(-5.61317670591776,-8.19170441954395,-70.2479860613005));
#8587=CARTESIAN_POINT('Ctrl Pts',(-5.74417600481268,-8.18935583496947,-70.3377118983739));
#8588=CARTESIAN_POINT('Ctrl Pts',(-5.87319237329383,-8.1869339839657,-70.4306632680959));
#8589=CARTESIAN_POINT('Ctrl Pts',(-6.00000000000001,-8.18443804034608,-70.5266968882262));
#8590=CARTESIAN_POINT('Ctrl Pts',(6.,-8.18443804034608,-70.5266968882262));
#8591=CARTESIAN_POINT('Ctrl Pts',(5.83935589890228,-8.1875999843835,-70.4050383178254));
#8592=CARTESIAN_POINT('Ctrl Pts',(5.67578673642156,-8.19064303069535,-70.2887847010274));
#8593=CARTESIAN_POINT('Ctrl Pts',(5.50942106147531,-8.19356119742072,-70.1778680148472));
#8594=CARTESIAN_POINT('Ctrl Pts',(5.34128427556694,-8.19651043063309,-70.0657705216355));
#8595=CARTESIAN_POINT('Ctrl Pts',(5.17029064779969,-8.19933205929434,-69.9591237634446));
#8596=CARTESIAN_POINT('Ctrl Pts',(4.99653358519068,-8.20202243644602,-69.8578934495407));
#8597=CARTESIAN_POINT('Ctrl Pts',(4.8804127072399,-8.20382040052403,-69.7902417941246));
#8598=CARTESIAN_POINT('Ctrl Pts',(4.76305682585017,-8.20555979931183,-69.7250099731657));
#8599=CARTESIAN_POINT('Ctrl Pts',(4.64448583892399,-8.20724032943103,-69.6621979344201));
#8600=CARTESIAN_POINT('Ctrl Pts',(4.48748709677556,-8.2094655037481,-69.5790290975023));
#8601=CARTESIAN_POINT('Ctrl Pts',(4.32836434918063,-8.21158809145558,-69.5001027126829));
#8602=CARTESIAN_POINT('Ctrl Pts',(4.16706106631021,-8.21360403193805,-69.4254068252458));
#8603=CARTESIAN_POINT('Ctrl Pts',(4.08612566398949,-8.21461554857367,-69.3879274783048));
#8604=CARTESIAN_POINT('Ctrl Pts',(4.00464093265679,-8.21560028549895,-69.351513944954));
#8605=CARTESIAN_POINT('Ctrl Pts',(3.92259791175199,-8.21655817297074,-69.3161692970076));
#8606=CARTESIAN_POINT('Ctrl Pts',(3.72085798171443,-8.21891357321577,-69.2292584699165));
#8607=CARTESIAN_POINT('Ctrl Pts',(3.515745117614,-8.22110667449109,-69.1488092724985));
#8608=CARTESIAN_POINT('Ctrl Pts',(3.30737505839146,-8.22311989481481,-69.0750285052789));
#8609=CARTESIAN_POINT('Ctrl Pts',(3.26212128379759,-8.22355712566783,-69.0590048106004));
#8610=CARTESIAN_POINT('Ctrl Pts',(3.21671388216392,-8.22398588824251,-69.0432958404281));
#8611=CARTESIAN_POINT('Ctrl Pts',(3.17115406088249,-8.22440602934023,-69.0279040399477));
#8612=CARTESIAN_POINT('Ctrl Pts',(3.04348452784257,-8.22558336534041,-68.9847725279113));
#8613=CARTESIAN_POINT('Ctrl Pts',(2.91461436345215,-8.22669344285102,-68.9441351923562));
#8614=CARTESIAN_POINT('Ctrl Pts',(2.784937514944,-8.2277368326506,-68.9061417077793));
#8615=CARTESIAN_POINT('Ctrl Pts',(2.65526066643585,-8.22878022245018,-68.8681482232025));
#8616=CARTESIAN_POINT('Ctrl Pts',(2.52477746828391,-8.22975694690195,-68.8327986930296));
#8617=CARTESIAN_POINT('Ctrl Pts',(2.39389751143945,-8.23066112223301,-68.8001908239837));
#8618=CARTESIAN_POINT('Ctrl Pts',(2.24586149903464,-8.23168381901373,-68.7633086380252));
#8619=CARTESIAN_POINT('Ctrl Pts',(2.09732185681607,-8.23261249774906,-68.7299245554918));
#8620=CARTESIAN_POINT('Ctrl Pts',(1.94812127075837,-8.23344107483214,-68.6999793435983));
#8621=CARTESIAN_POINT('Ctrl Pts',(1.83350272325276,-8.23407760250451,-68.6769748984907));
#8622=CARTESIAN_POINT('Ctrl Pts',(1.71849372454123,-8.23465515294992,-68.6560009217279));
#8623=CARTESIAN_POINT('Ctrl Pts',(1.6030186314804,-8.2351730392858,-68.6370508939283));
#8624=CARTESIAN_POINT('Ctrl Pts',(1.44517413123055,-8.23588094527407,-68.6111478390924));
#8625=CARTESIAN_POINT('Ctrl Pts',(1.28644990400479,-8.23647732620875,-68.589032311698));
#8626=CARTESIAN_POINT('Ctrl Pts',(1.12724839634008,-8.23697240718817,-68.5707819182047));
#8627=CARTESIAN_POINT('Ctrl Pts',(0.96806767754036,-8.23746742351888,-68.5525339078858));
#8628=CARTESIAN_POINT('Ctrl Pts',(0.808410173874957,-8.23786117621294,-68.5381500692541));
#8629=CARTESIAN_POINT('Ctrl Pts',(0.648684626042312,-8.23815664722233,-68.5276567709296));
#8630=CARTESIAN_POINT('Ctrl Pts',(0.488781786876221,-8.2384524461971,-68.5171518253084));
#8631=CARTESIAN_POINT('Ctrl Pts',(0.328811127110583,-8.23864974756345,-68.5105460654646));
#8632=CARTESIAN_POINT('Ctrl Pts',(0.169183612391038,-8.23874419313204,-68.5078142233184));
#8633=CARTESIAN_POINT('Ctrl Pts',(0.112740170955557,-8.2387775885835,-68.5068482584441));
#8634=CARTESIAN_POINT('Ctrl Pts',(0.0563396137314528,-8.23879805702532,
-68.5063661755286));
#8635=CARTESIAN_POINT('Ctrl Pts',(-7.6571373978539E-15,-8.23880518655807,
-68.5063653181071));
#8636=CARTESIAN_POINT('Ctrl Pts',(-1.22464679914735E-15,-68.5063652081765,
-8.23880610063971));
#8637=CARTESIAN_POINT('Ctrl Pts',(0.00143095575713891,-68.5063652134009,
-8.23880605719895));
#8638=CARTESIAN_POINT('Ctrl Pts',(0.00286193022978105,-68.5063655290304,
-8.23880600505331));
#8639=CARTESIAN_POINT('Ctrl Pts',(0.00429292337380016,-68.5063661550895,
-8.23880594420307));
#8640=CARTESIAN_POINT('Ctrl Pts',(0.139173304405083,-68.5064251652143,-8.23880020867207));
#8641=CARTESIAN_POINT('Ctrl Pts',(0.274219837871558,-68.5092463995564,-8.23871827360899));
#8642=CARTESIAN_POINT('Ctrl Pts',(0.409024941780786,-68.5148232638019,-8.2385633499616));
#8643=CARTESIAN_POINT('Ctrl Pts',(0.543830045690013,-68.5204001280475,-8.23840842631422));
#8644=CARTESIAN_POINT('Ctrl Pts',(0.678393385609739,-68.528732587766,-8.2381805078804));
#8645=CARTESIAN_POINT('Ctrl Pts',(0.812310796291931,-68.5397620635481,-8.23787599113737));
#8646=CARTESIAN_POINT('Ctrl Pts',(0.981838135137693,-68.5537243830754,-8.23749050046207));
#8647=CARTESIAN_POINT('Ctrl Pts',(1.15033458376048,-68.5719977907132,-8.23698101142716));
#8648=CARTESIAN_POINT('Ctrl Pts',(1.31789673537818,-68.5945103285804,-8.23635430529869));
#8649=CARTESIAN_POINT('Ctrl Pts',(1.41506462229892,-68.6075651605497,-8.23599088366895));
#8650=CARTESIAN_POINT('Ctrl Pts',(1.5119184072392,-68.6220464790647,-8.23558813775747));
#8651=CARTESIAN_POINT('Ctrl Pts',(1.60847689897075,-68.6379482314015,-8.23514815153247));
#8652=CARTESIAN_POINT('Ctrl Pts',(1.78446273565371,-68.6669304901292,-8.23434624025003));
#8653=CARTESIAN_POINT('Ctrl Pts',(1.9594583758023,-68.7006270056341,-8.23341922375072));
#8654=CARTESIAN_POINT('Ctrl Pts',(2.1335183778158,-68.7390365074673,-8.23236162604042));
#8655=CARTESIAN_POINT('Ctrl Pts',(2.30698468192499,-68.7773149990713,-8.23130763566975));
#8656=CARTESIAN_POINT('Ctrl Pts',(2.47952223308019,-68.8202745200974,-8.23012397391906));
#8657=CARTESIAN_POINT('Ctrl Pts',(2.65117268232151,-68.8679636632795,-8.22880952393426));
#8658=CARTESIAN_POINT('Ctrl Pts',(2.82221883563617,-68.9154849166886,-8.22749970147462));
#8659=CARTESIAN_POINT('Ctrl Pts',(2.99238462345483,-68.9677027089631,-8.22606003552361));
#8660=CARTESIAN_POINT('Ctrl Pts',(3.16169140425706,-69.0247124774534,-8.22449335732444));
#8661=CARTESIAN_POINT('Ctrl Pts',(3.28911594250015,-69.0676194619865,-8.22331423593804));
#8662=CARTESIAN_POINT('Ctrl Pts',(3.41605288753761,-69.1132483787518,-8.22206469909378));
#8663=CARTESIAN_POINT('Ctrl Pts',(3.54205396079164,-69.1614646919926,-8.22075210685047));
#8664=CARTESIAN_POINT('Ctrl Pts',(3.66805503404568,-69.2096810052334,-8.21943951460716));
#8665=CARTESIAN_POINT('Ctrl Pts',(3.79311985917955,-69.2604845808539,-8.21806383776203));
#8666=CARTESIAN_POINT('Ctrl Pts',(3.91682185879893,-69.3136831042134,-8.21662552408077));
#8667=CARTESIAN_POINT('Ctrl Pts',(4.08469785324958,-69.385878824895,-8.21467358845874));
#8668=CARTESIAN_POINT('Ctrl Pts',(4.25007336704315,-69.4624744124128,-8.21260495076621));
#8669=CARTESIAN_POINT('Ctrl Pts',(4.41300814181022,-69.5434155490575,-8.21042789515496));
#8670=CARTESIAN_POINT('Ctrl Pts',(4.49019533936177,-69.5817598467261,-8.20939655717456));
#8671=CARTESIAN_POINT('Ctrl Pts',(4.5668345824311,-69.621080106923,-8.20834096177747));
#8672=CARTESIAN_POINT('Ctrl Pts',(4.64293089072211,-69.6613743873479,-8.20726237441504));
#8673=CARTESIAN_POINT('Ctrl Pts',(4.8103442668302,-69.750022597429,-8.20488946098699));
#8674=CARTESIAN_POINT('Ctrl Pts',(4.97512450913361,-69.8433787748153,-8.20240389161162));
#8675=CARTESIAN_POINT('Ctrl Pts',(5.13727477281679,-69.9414411800462,-8.19980502327808));
#8676=CARTESIAN_POINT('Ctrl Pts',(5.29870860352638,-70.0390703134527,-8.19721763759604));
#8677=CARTESIAN_POINT('Ctrl Pts',(5.45753612340623,-70.1413645072354,-8.19451799482584));
#8678=CARTESIAN_POINT('Ctrl Pts',(5.6137317611851,-70.2483645458481,-8.19170920857795));
#8679=CARTESIAN_POINT('Ctrl Pts',(5.74433956218909,-70.3378359289754,-8.18936055530861));
#8680=CARTESIAN_POINT('Ctrl Pts',(5.87310679411424,-70.4305984731283,-8.18693566805311));
#8681=CARTESIAN_POINT('Ctrl Pts',(5.99999937459725,-70.5266964145979,-8.18443805265555));
#8682=CARTESIAN_POINT('Ctrl Pts',(5.9999983295249,-70.5266991009391,8.18443799239331));
#8683=CARTESIAN_POINT('Ctrl Pts',(5.86952914135541,-70.4279042693595,8.18700573286285));
#8684=CARTESIAN_POINT('Ctrl Pts',(5.73648042273753,-70.3322021606331,8.1895046414597));
#8685=CARTESIAN_POINT('Ctrl Pts',(5.60141216089113,-70.2399589008432,8.19192377023309));
#8686=CARTESIAN_POINT('Ctrl Pts',(5.53449126469586,-70.1942560722976,8.19312235133062));
#8687=CARTESIAN_POINT('Ctrl Pts',(5.46707376398794,-70.1494025624782,8.19430134521795));
#8688=CARTESIAN_POINT('Ctrl Pts',(5.39922360708421,-70.1054449275604,8.19545938490334));
#8689=CARTESIAN_POINT('Ctrl Pts',(5.25743408344076,-70.0135846813957,8.19787939250308));
#8690=CARTESIAN_POINT('Ctrl Pts',(5.11375652902179,-69.9256335512281,8.20020796766627));
#8691=CARTESIAN_POINT('Ctrl Pts',(4.96827129693732,-69.841514422138,8.20244556438375));
#8692=CARTESIAN_POINT('Ctrl Pts',(4.87803597365184,-69.7893406262195,8.20383340464968));
#8693=CARTESIAN_POINT('Ctrl Pts',(4.78710469185803,-69.7386418773235,8.20518622571968));
#8694=CARTESIAN_POINT('Ctrl Pts',(4.69549237430863,-69.6894088764903,8.20650391776634));
#8695=CARTESIAN_POINT('Ctrl Pts',(4.6762564686983,-69.6790713871409,8.2067805945333));
#8696=CARTESIAN_POINT('Ctrl Pts',(4.65699052868404,-69.6687985443116,8.20705572191943));
#8697=CARTESIAN_POINT('Ctrl Pts',(4.63769388209867,-69.6585901039548,8.20732930453224));
#8698=CARTESIAN_POINT('Ctrl Pts',(4.39017962767364,-69.5276484663706,8.21083849438733));
#8699=CARTESIAN_POINT('Ctrl Pts',(4.13833520205855,-69.4076810004414,8.2140751261655));
#8700=CARTESIAN_POINT('Ctrl Pts',(3.88172272152124,-69.2985071798683,8.21703503037178));
#8701=CARTESIAN_POINT('Ctrl Pts',(3.66073824435755,-69.2044910213058,8.21958398232497));
#8702=CARTESIAN_POINT('Ctrl Pts',(3.43621759575504,-69.1184802024722,8.22192769806047));
#8703=CARTESIAN_POINT('Ctrl Pts',(3.20786877787091,-69.040387840584,8.2240628011651));
#8704=CARTESIAN_POINT('Ctrl Pts',(3.19424339780753,-69.0357281356614,8.22419020095435));
#8705=CARTESIAN_POINT('Ctrl Pts',(3.18060438420692,-69.0310966313511,8.22431685779488));
#8706=CARTESIAN_POINT('Ctrl Pts',(3.16695192959349,-69.0264934493831,8.22444276748959));
#8707=CARTESIAN_POINT('Ctrl Pts',(2.95485023303377,-68.95497937132,8.22639887433025));
#8708=CARTESIAN_POINT('Ctrl Pts',(2.73944418113102,-68.8902852528574,8.22817652038379));
#8709=CARTESIAN_POINT('Ctrl Pts',(2.52171858644569,-68.8329431873267,8.22975681571581));
#8710=CARTESIAN_POINT('Ctrl Pts',(2.48914750906238,-68.8243649911968,8.22999322302301));
#8711=CARTESIAN_POINT('Ctrl Pts',(2.4565245579048,-68.8159512403314,8.23022521610616));
#8712=CARTESIAN_POINT('Ctrl Pts',(2.42385306368375,-68.8077036207449,8.23045273427335));
#8713=CARTESIAN_POINT('Ctrl Pts',(2.41330752868356,-68.8050414969856,8.23052617140418));
#8714=CARTESIAN_POINT('Ctrl Pts',(2.40275693634491,-68.8023966811721,8.23059914232783));
#8715=CARTESIAN_POINT('Ctrl Pts',(2.39220145545524,-68.7997691986063,8.2306716459234));
#8716=CARTESIAN_POINT('Ctrl Pts',(2.15048775697385,-68.739601543971,8.23233193145869));
#8717=CARTESIAN_POINT('Ctrl Pts',(1.90618545878813,-68.6885125030794,8.23374612624222));
#8718=CARTESIAN_POINT('Ctrl Pts',(1.66089102088927,-68.6467302669797,8.23490402309128));
#8719=CARTESIAN_POINT('Ctrl Pts',(1.64754851003194,-68.6444575699566,8.23496700556823));
#8720=CARTESIAN_POINT('Ctrl Pts',(1.63420306192931,-68.6422124215772,8.23502922939213));
#8721=CARTESIAN_POINT('Ctrl Pts',(1.62085493312774,-68.6399948629774,8.23509069279914));
#8722=CARTESIAN_POINT('Ctrl Pts',(1.61374908486424,-68.6388143503259,8.23512341271445));
#8723=CARTESIAN_POINT('Ctrl Pts',(1.60664247690719,-68.637641656468,8.23515591713173));
#8724=CARTESIAN_POINT('Ctrl Pts',(1.59953508414201,-68.6364767804816,8.23518820602338));
#8725=CARTESIAN_POINT('Ctrl Pts',(1.33718455630123,-68.5934784771657,8.23638006470422));
#8726=CARTESIAN_POINT('Ctrl Pts',(1.07384822645327,-68.5611469627105,8.23728059896383));
#8727=CARTESIAN_POINT('Ctrl Pts',(0.808525090100186,-68.539451008081,8.23788453741318));
#8728=CARTESIAN_POINT('Ctrl Pts',(0.804925810356564,-68.5391566884408,8.23789273022839));
#8729=CARTESIAN_POINT('Ctrl Pts',(0.801326165025958,-68.538864325773,8.23790086846902));
#8730=CARTESIAN_POINT('Ctrl Pts',(0.797726162962058,-68.5385739203607,8.23790895211685));
#8731=CARTESIAN_POINT('Ctrl Pts',(0.532630993747636,-68.5171891904231,8.23850421177229));
#8732=CARTESIAN_POINT('Ctrl Pts',(0.265540661321849,-68.5064142752162,8.23880459800998));
#8733=CARTESIAN_POINT('Ctrl Pts',(-3.51073400206478E-10,-68.5063672600388,
8.23880581768755));
#8734=CARTESIAN_POINT('',(6.00000000000001,-8.18443804034558,70.5266968882263));
#8735=CARTESIAN_POINT('Ctrl Pts',(4.16541472538293E-10,-8.23880590935122,
68.5063673993548));
#8736=CARTESIAN_POINT('Ctrl Pts',(0.00416345598546408,-8.23880592987024,
68.506366666553));
#8737=CARTESIAN_POINT('Ctrl Pts',(0.277610744887515,-8.23880245316255,68.5064915939776));
#8738=CARTESIAN_POINT('Ctrl Pts',(0.816727761679238,-8.23816650019571,68.5293033513698));
#8739=CARTESIAN_POINT('Ctrl Pts',(1.61170598678262,-8.23543318022081,68.6275793681561));
#8740=CARTESIAN_POINT('Ctrl Pts',(2.39732558377894,-8.23094391608953,68.7897189261084));
#8741=CARTESIAN_POINT('Ctrl Pts',(3.17804312806208,-8.22465018744083,69.0185952328547));
#8742=CARTESIAN_POINT('Ctrl Pts',(3.92894292458085,-8.21678502129265,69.3072164748245));
#8743=CARTESIAN_POINT('Ctrl Pts',(4.89068866338157,-8.20435137693732,69.768539148429));
#8744=CARTESIAN_POINT('Ctrl Pts',(5.56837676918829,-8.19293364330735,70.1998211121876));
#8745=CARTESIAN_POINT('Ctrl Pts',(6.00000000000001,-8.18443804034558,70.5266968882263));
#8746=CARTESIAN_POINT('',(6.00000079446281,8.18443781970293,70.5266943053403));
#8747=CARTESIAN_POINT('Origin',(6.,0.,0.));
#8748=CARTESIAN_POINT('Ctrl Pts',(6.00000079446281,8.18443781970294,70.5266943053403));
#8749=CARTESIAN_POINT('Ctrl Pts',(5.82155183841513,8.18794923220616,70.3915366584588));
#8750=CARTESIAN_POINT('Ctrl Pts',(5.63916240398924,8.19132108429475,70.2627665326567));
#8751=CARTESIAN_POINT('Ctrl Pts',(5.45240408670687,8.1945511670375,70.1401258483009));
#8752=CARTESIAN_POINT('Ctrl Pts',(5.43621847707622,8.1948311056186,70.1294970620134));
#8753=CARTESIAN_POINT('Ctrl Pts',(5.42000008376334,8.1951099797053,70.118914304163));
#8754=CARTESIAN_POINT('Ctrl Pts',(5.40374864585165,8.19538778805092,70.1083774012658));
#8755=CARTESIAN_POINT('Ctrl Pts',(5.38105594658528,8.19577570580165,70.0936641943519));
#8756=CARTESIAN_POINT('Ctrl Pts',(5.35829881879662,8.19616154554046,70.0790403964617));
#8757=CARTESIAN_POINT('Ctrl Pts',(5.33548081285126,8.19654524000997,70.0645079277786));
#8758=CARTESIAN_POINT('Ctrl Pts',(5.18185112519004,8.19912858851329,69.9666633295222));
#8759=CARTESIAN_POINT('Ctrl Pts',(5.02530020323893,8.20161758690385,69.8728510426696));
#8760=CARTESIAN_POINT('Ctrl Pts',(4.8666174970433,8.20399815192714,69.7835350039511));
#8761=CARTESIAN_POINT('Ctrl Pts',(4.81060345528634,8.20483847707547,69.7520069789867));
#8762=CARTESIAN_POINT('Ctrl Pts',(4.75432336621731,8.20566528575196,69.7210394644626));
#8763=CARTESIAN_POINT('Ctrl Pts',(4.69781078689656,8.20647793764918,69.6906538318512));
#8764=CARTESIAN_POINT('Ctrl Pts',(4.67712257658307,8.20677543448199,69.6795302136139));
#8765=CARTESIAN_POINT('Ctrl Pts',(4.65640320427027,8.20707103395485,69.6684845823009));
#8766=CARTESIAN_POINT('Ctrl Pts',(4.63565284037979,8.20736473752302,69.6575167460913));
#8767=CARTESIAN_POINT('Ctrl Pts',(4.46538751060781,8.20977469694131,69.5675211075104));
#8768=CARTESIAN_POINT('Ctrl Pts',(4.29313372624732,8.21205392334671,69.4828105614274));
#8769=CARTESIAN_POINT('Ctrl Pts',(4.11901696281379,8.21420099130811,69.4033085084354));
#8770=CARTESIAN_POINT('Ctrl Pts',(4.06713153073576,8.21484080074794,69.3796175191864));
#8771=CARTESIAN_POINT('Ctrl Pts',(4.01508053132934,8.21546886660144,69.3563893661196));
#8772=CARTESIAN_POINT('Ctrl Pts',(3.96286696914459,8.21608513032504,69.3336228546209));
#8773=CARTESIAN_POINT('Ctrl Pts',(3.94536666907604,8.21629168202604,69.3259922550972));
#8774=CARTESIAN_POINT('Ctrl Pts',(3.92784810612159,8.21649690782433,69.318413518385));
#8775=CARTESIAN_POINT('Ctrl Pts',(3.91031105586775,8.21670080821778,69.3108865238576));
#8776=CARTESIAN_POINT('Ctrl Pts',(3.67860897710432,8.21939477010644,69.2114387687571));
#8777=CARTESIAN_POINT('Ctrl Pts',(3.44372375805669,8.22185815037421,69.1210462160137));
#8778=CARTESIAN_POINT('Ctrl Pts',(3.20575717391094,8.22408401789359,69.0396653507124));
#8779=CARTESIAN_POINT('Ctrl Pts',(3.19164154379547,8.22421605123223,69.0348380250726));
#8780=CARTESIAN_POINT('Ctrl Pts',(3.17751507598537,8.22434724919125,69.0300423949384));
#8781=CARTESIAN_POINT('Ctrl Pts',(3.16337770078198,8.22447760976305,69.0252784817195));
#8782=CARTESIAN_POINT('Ctrl Pts',(2.9211665930845,8.22671103556112,68.9436598869558));
#8783=CARTESIAN_POINT('Ctrl Pts',(2.67577731324865,8.2286990141984,68.8713564483493));
#8784=CARTESIAN_POINT('Ctrl Pts',(2.42661791252754,8.23043466497516,68.808401884732));
#8785=CARTESIAN_POINT('Ctrl Pts',(2.41606416224099,8.23050818267038,68.8057352916117));
#8786=CARTESIAN_POINT('Ctrl Pts',(2.40550364625273,8.23058124754378,68.8030854757963));
#8787=CARTESIAN_POINT('Ctrl Pts',(2.39493649585478,8.23065385797032,68.8004524833151));
#8788=CARTESIAN_POINT('Ctrl Pts',(2.14155816613234,8.23239490526352,68.7373187895628));
#8789=CARTESIAN_POINT('Ctrl Pts',(1.88427006063706,8.23387456206401,68.6838391773228));
#8790=CARTESIAN_POINT('Ctrl Pts',(1.62517257027932,8.23507095393907,68.6407124984445));
#8791=CARTESIAN_POINT('Ctrl Pts',(1.61835756045793,8.23510242248926,68.6395781426478));
#8792=CARTESIAN_POINT('Ctrl Pts',(1.61154129987145,8.23513369515959,68.6384509459718));
#8793=CARTESIAN_POINT('Ctrl Pts',(1.60472381969236,8.23516477189413,68.6373309098572));
#8794=CARTESIAN_POINT('Ctrl Pts',(1.34152296839364,8.23636454406381,68.5940899394226));
#8795=CARTESIAN_POINT('Ctrl Pts',(1.0765164340326,8.23727044669812,68.561520555236));
#8796=CARTESIAN_POINT('Ctrl Pts',(0.81117025799267,8.23787819074675,68.5396682419934));
#8797=CARTESIAN_POINT('Ctrl Pts',(0.808339331029581,8.2378846746503,68.5394351038955));
#8798=CARTESIAN_POINT('Ctrl Pts',(0.80550836537592,8.23789112460624,68.5392031860196));
#8799=CARTESIAN_POINT('Ctrl Pts',(0.802677360020277,8.23789754061042,68.5389724884737));
#8800=CARTESIAN_POINT('Ctrl Pts',(0.53568415341721,8.23850263643787,68.5172153139734));
#8801=CARTESIAN_POINT('Ctrl Pts',(0.268362014995775,8.23880636303395,68.5063145889559));
#8802=CARTESIAN_POINT('Ctrl Pts',(-2.38940450967676E-10,8.23880549026604,
68.5063639612443));
#8803=CARTESIAN_POINT('Ctrl Pts',(-8.95159733014031E-12,68.5063647597673,
8.23880598322944));
#8804=CARTESIAN_POINT('Ctrl Pts',(0.000821623443402016,68.5063649144486,
8.23880597887183));
#8805=CARTESIAN_POINT('Ctrl Pts',(0.271041635589146,68.5064494487375,8.2388036071868));
#8806=CARTESIAN_POINT('Ctrl Pts',(0.813049986647028,68.5287264288495,8.23818246295993));
#8807=CARTESIAN_POINT('Ctrl Pts',(1.87711179906711,68.6604780686295,8.23451866590537));
#8808=CARTESIAN_POINT('Ctrl Pts',(2.91023424206843,68.9172079362927,8.22741504885044));
#8809=CARTESIAN_POINT('Ctrl Pts',(3.9186730012011,69.3024856616359,8.216912881982));
#8810=CARTESIAN_POINT('Ctrl Pts',(4.89035765134611,69.7679092313649,8.20436742745112));
#8811=CARTESIAN_POINT('Ctrl Pts',(5.56902654677854,70.2003132763431,8.1929208520031));
#8812=CARTESIAN_POINT('Ctrl Pts',(5.99999909300179,70.5266962013408,8.18443805819819));
#8813=CARTESIAN_POINT('Ctrl Pts',(5.99999728414902,70.526700485917,-8.18443796047155));
#8814=CARTESIAN_POINT('Ctrl Pts',(5.88877062295712,70.4424830590272,-8.18662683690695));
#8815=CARTESIAN_POINT('Ctrl Pts',(5.77574490007538,70.3605798226138,-8.18876497800162));
#8816=CARTESIAN_POINT('Ctrl Pts',(5.66125555859731,70.2811701233984,-8.19084582792973));
#8817=CARTESIAN_POINT('Ctrl Pts',(5.57445682198249,70.2209666015868,-8.19242339962779));
#8818=CARTESIAN_POINT('Ctrl Pts',(5.48681542965758,70.1621965864257,-8.19396803945737));
#8819=CARTESIAN_POINT('Ctrl Pts',(5.39846309902672,70.104951809959,-8.19547660000369));
#8820=CARTESIAN_POINT('Ctrl Pts',(5.37712412501396,70.091125974368,-8.19584094958071));
#8821=CARTESIAN_POINT('Ctrl Pts',(5.3557436421719,70.0773891765976,-8.19620319302142));
#8822=CARTESIAN_POINT('Ctrl Pts',(5.33431990260324,70.0637400838969,-8.19656335494725));
#8823=CARTESIAN_POINT('Ctrl Pts',(5.12555734430554,69.9307371830023,-8.20007293481291));
#8824=CARTESIAN_POINT('Ctrl Pts',(4.91298617423999,69.8062578101768,-8.20338216870485));
#8825=CARTESIAN_POINT('Ctrl Pts',(4.6966209436992,69.6900147108326,-8.20649206551354));
#8826=CARTESIAN_POINT('Ctrl Pts',(4.67758612395171,69.6797881765721,-8.20676565995863));
#8827=CARTESIAN_POINT('Ctrl Pts',(4.65852195332554,69.6696253597668,-8.20703771231119));
#8828=CARTESIAN_POINT('Ctrl Pts',(4.63942867597594,69.6595263429874,-8.20730821675026));
#8829=CARTESIAN_POINT('Ctrl Pts',(4.41919463829539,69.5430378428103,-8.21042838746465));
#8830=CARTESIAN_POINT('Ctrl Pts',(4.1948631000602,69.4349201743698,-8.21334228193345));
#8831=CARTESIAN_POINT('Ctrl Pts',(3.9666611220002,69.3352782563471,-8.21603993954926));
#8832=CARTESIAN_POINT('Ctrl Pts',(3.71881052821058,69.2270569834282,-8.21896987051482));
#8833=CARTESIAN_POINT('Ctrl Pts',(3.46639444521359,69.128834043849,-8.22164471824023));
#8834=CARTESIAN_POINT('Ctrl Pts',(3.20863192391708,69.0406490402862,-8.22405548872155));
#8835=CARTESIAN_POINT('Ctrl Pts',(3.1948218931075,69.0359243905969,-8.22418464952606));
#8836=CARTESIAN_POINT('Ctrl Pts',(3.18099651671809,69.0312285512257,-8.22431305238602));
#8837=CARTESIAN_POINT('Ctrl Pts',(3.16715627968411,69.0265616991943,-8.22444069139633));
#8838=CARTESIAN_POINT('Ctrl Pts',(2.92272573864455,68.9441410611525,-8.2266949065714));
#8839=CARTESIAN_POINT('Ctrl Pts',(2.67368605348898,68.8707694212835,-8.22871285737206));
#8840=CARTESIAN_POINT('Ctrl Pts',(2.42264702829873,68.8073992448633,-8.23046107662634));
#8841=CARTESIAN_POINT('Ctrl Pts',(2.41178473411857,68.8046572588394,-8.23053672092832));
#8842=CARTESIAN_POINT('Ctrl Pts',(2.4009186965982,68.8019339994299,-8.23061186018697));
#8843=CARTESIAN_POINT('Ctrl Pts',(2.3900489422933,68.7992294611676,-8.23068649406848));
#8844=CARTESIAN_POINT('Ctrl Pts',(2.13547959455546,68.7358892492317,-8.23243441752685));
#8845=CARTESIAN_POINT('Ctrl Pts',(1.87896849200073,68.6828384134398,-8.23390321081528));
#8846=CARTESIAN_POINT('Ctrl Pts',(1.62076868896401,68.6399805175378,-8.2350913428248));
#8847=CARTESIAN_POINT('Ctrl Pts',(1.61314971826133,68.6387158649338,-8.23512640227436));
#8848=CARTESIAN_POINT('Ctrl Pts',(1.60552927668701,68.6374600903476,-8.23516121726959));
#8849=CARTESIAN_POINT('Ctrl Pts',(1.59790736495981,68.6362131981471,-8.23519578763072));
#8850=CARTESIAN_POINT('Ctrl Pts',(1.33624255857368,68.5934066401744,-8.23638260888731));
#8851=CARTESIAN_POINT('Ctrl Pts',(1.07285116140782,68.5610718339649,-8.23728255736077));
#8852=CARTESIAN_POINT('Ctrl Pts',(0.807971934124623,68.5394056876693,-8.23788571950343));
#8853=CARTESIAN_POINT('Ctrl Pts',(0.803663067258854,68.5390532382121,-8.23789553131615));
#8854=CARTESIAN_POINT('Ctrl Pts',(0.799353806765366,68.5387036113629,-8.23790526460795));
#8855=CARTESIAN_POINT('Ctrl Pts',(0.795044166515618,68.53835680702,-8.23791491937101));
#8856=CARTESIAN_POINT('Ctrl Pts',(0.530457939610201,68.5170650872393,-8.23850766428316));
#8857=CARTESIAN_POINT('Ctrl Pts',(0.264393140237664,68.5064088475944,-8.23880474753574));
#8858=CARTESIAN_POINT('Ctrl Pts',(-2.73511885838946E-10,68.5063670000441,
-8.23880582348961));
#8859=CARTESIAN_POINT('Ctrl Pts',(-3.18401114664506E-12,8.23880597151339,
-68.5063651759543));
#8860=CARTESIAN_POINT('Ctrl Pts',(0.000197208001215656,8.23880597105813,
-68.5063651919466));
#8861=CARTESIAN_POINT('Ctrl Pts',(0.269379031644614,8.23880512607218,-68.5063950399915));
#8862=CARTESIAN_POINT('Ctrl Pts',(0.808562402718581,8.23819328895472,-68.5283381860597));
#8863=CARTESIAN_POINT('Ctrl Pts',(1.87925012401009,8.23451686535867,-68.6605385446451));
#8864=CARTESIAN_POINT('Ctrl Pts',(2.91199036992062,8.22738994814212,-68.9181356819889));
#8865=CARTESIAN_POINT('Ctrl Pts',(3.9138431051418,8.21696851242034,-69.3004357176585));
#8866=CARTESIAN_POINT('Ctrl Pts',(4.89022818173288,8.20437701925203,-69.7675337025404));
#8867=CARTESIAN_POINT('Ctrl Pts',(5.56909800240238,8.19291944450744,-70.2003674353596));
#8868=CARTESIAN_POINT('Ctrl Pts',(5.99999856012047,8.18443806868659,-70.5266957977807));
#8869=CARTESIAN_POINT('Origin',(6.,-81.,6.));
#8870=CARTESIAN_POINT('Origin',(6.,0.,0.));
#8871=CARTESIAN_POINT('Ctrl Pts',(6.,6.00000000000024,68.1397368351434));
#8872=CARTESIAN_POINT('Ctrl Pts',(6.,6.00000000000025,68.4372608978003));
#8873=CARTESIAN_POINT('Ctrl Pts',(6.,6.04965101665905,68.7349461355828));
#8874=CARTESIAN_POINT('Ctrl Pts',(6.,6.2446302212969,69.3064823965443));
#8875=CARTESIAN_POINT('Ctrl Pts',(6.00000000000135,6.39328919939164,69.5806121655312));
#8876=CARTESIAN_POINT('Ctrl Pts',(6.00000000000135,6.76208224766943,70.0282007545523));
#8877=CARTESIAN_POINT('Ctrl Pts',(6.,6.9733548679495,70.2089295378112));
#8878=CARTESIAN_POINT('Ctrl Pts',(6.,7.37004430436642,70.4192718977462));
#8879=CARTESIAN_POINT('Ctrl Pts',(5.99999999998631,7.53536956523719,70.4786001966803));
#8880=CARTESIAN_POINT('Ctrl Pts',(5.99999999998631,7.86537303383998,70.5396271940705));
#8881=CARTESIAN_POINT('Ctrl Pts',(6.,8.02526185723979,70.5451663805613));
#8882=CARTESIAN_POINT('Ctrl Pts',(6.,8.18443767292577,70.5266937224604));
#8883=CARTESIAN_POINT('Ctrl Pts',(6.,-8.1844379396224,70.5267011803182));
#8884=CARTESIAN_POINT('Ctrl Pts',(6.,-8.0258764476141,70.5451008684421));
#8885=CARTESIAN_POINT('Ctrl Pts',(6.00000000003114,-7.86660084437536,70.5396767302592));
#8886=CARTESIAN_POINT('Ctrl Pts',(6.00000000003114,-7.53785118706882,70.4792699334571));
#8887=CARTESIAN_POINT('Ctrl Pts',(6.,-7.37311003018443,70.4204832009684));
#8888=CARTESIAN_POINT('Ctrl Pts',(6.,-6.97693717792651,70.2115400596563));
#8889=CARTESIAN_POINT('Ctrl Pts',(6.00000000000216,-6.76557809943801,70.0315615011381));
#8890=CARTESIAN_POINT('Ctrl Pts',(6.00000000000216,-6.39627772637684,69.5853535340167));
#8891=CARTESIAN_POINT('Ctrl Pts',(6.,-6.24722968116823,69.3118720006602));
#8892=CARTESIAN_POINT('Ctrl Pts',(6.,-6.05037840315953,68.7391559470898));
#8893=CARTESIAN_POINT('Ctrl Pts',(6.,-6.00000402839798,68.4393237078532));
#8894=CARTESIAN_POINT('Ctrl Pts',(6.,-6.00000000024154,68.1396788547224));
#8895=CARTESIAN_POINT('Origin',(-6.,81.,6.));
#8896=CARTESIAN_POINT('Origin',(-6.,1.17789865652746E-16,0.));
#8897=CARTESIAN_POINT('Ctrl Pts',(-6.,68.1397019025295,6.00000000000004));
#8898=CARTESIAN_POINT('Ctrl Pts',(-6.,68.4372486108155,5.99999994767389));
#8899=CARTESIAN_POINT('Ctrl Pts',(-6.,68.734965697874,6.0496595769299));
#8900=CARTESIAN_POINT('Ctrl Pts',(-6.,69.3065130464615,6.24464436565585));
#8901=CARTESIAN_POINT('Ctrl Pts',(-6.00000000000061,69.580625839489,6.39329137641111));
#8902=CARTESIAN_POINT('Ctrl Pts',(-6.00000000000061,70.028203763518,6.76207415119899));
#8903=CARTESIAN_POINT('Ctrl Pts',(-6.00000000027369,70.208928253055,6.97334472427177));
#8904=CARTESIAN_POINT('Ctrl Pts',(-6.00000000027369,70.4192699121286,7.37003273462433));
#8905=CARTESIAN_POINT('Ctrl Pts',(-5.99999999998997,70.4785993003653,7.53536040161822));
#8906=CARTESIAN_POINT('Ctrl Pts',(-5.99999999998997,70.5396278066748,7.86536832103549));
#8907=CARTESIAN_POINT('Ctrl Pts',(-6.,70.5451673858303,8.02525949965797));
#8908=CARTESIAN_POINT('Ctrl Pts',(-6.,70.5266946612721,8.18443778189399));
#8909=CARTESIAN_POINT('Ctrl Pts',(-6.,70.5267027901716,-8.18443790289761));
#8910=CARTESIAN_POINT('Ctrl Pts',(-6.,70.5451026280608,-8.02587206439152));
#8911=CARTESIAN_POINT('Ctrl Pts',(-6.00000000004388,70.5396777866917,-7.86659240106826));
#8912=CARTESIAN_POINT('Ctrl Pts',(-6.00000000004388,70.4792681383387,-7.53783505312272));
#8913=CARTESIAN_POINT('Ctrl Pts',(-6.,70.4204793555461,-7.37308992300955));
#8914=CARTESIAN_POINT('Ctrl Pts',(-6.,70.2115359913312,-6.97692019146415));
#8915=CARTESIAN_POINT('Ctrl Pts',(-6.00000000000371,70.0315643000756,-6.76556755522217));
#8916=CARTESIAN_POINT('Ctrl Pts',(-6.00000000000371,69.5853654206441,-6.3962796681645));
#8917=CARTESIAN_POINT('Ctrl Pts',(-6.,69.3118877775374,-6.24723921228693));
#8918=CARTESIAN_POINT('Ctrl Pts',(-6.,68.739178955923,-6.05038425472732));
#8919=CARTESIAN_POINT('Ctrl Pts',(-6.,68.439335921525,-6.00000474549972));
#8920=CARTESIAN_POINT('Ctrl Pts',(-6.,68.1396788547224,-6.00000000033548));
#8921=CARTESIAN_POINT('Origin',(10.,0.,0.));
#8922=CARTESIAN_POINT('',(-10.,0.,-16.));
#8923=CARTESIAN_POINT('Origin',(-10.,0.,0.));
#8924=CARTESIAN_POINT('',(-8.,-1.95943487863577E-15,-16.));
#8925=CARTESIAN_POINT('',(10.,-1.95943487863577E-15,-16.));
#8926=CARTESIAN_POINT('Origin',(-8.,0.,0.));
#8927=CARTESIAN_POINT('',(8.,-1.95943487863577E-15,-16.));
#8928=CARTESIAN_POINT('Origin',(8.,0.,0.));
#8929=CARTESIAN_POINT('',(10.,0.,-16.));
#8930=CARTESIAN_POINT('',(10.,-1.95943487863577E-15,-16.));
#8931=CARTESIAN_POINT('Origin',(10.,0.,0.));
#8932=CARTESIAN_POINT('Origin',(8.,0.,0.));
#8933=CARTESIAN_POINT('Origin',(-8.,0.,0.));
#8934=CARTESIAN_POINT('Origin',(8.,0.,0.));
#8935=CARTESIAN_POINT('Origin',(-8.,0.,0.));
#8936=CARTESIAN_POINT('Origin',(8.,0.,0.));
#8937=CARTESIAN_POINT('Origin',(-8.,0.,0.));
#8938=CARTESIAN_POINT('Origin',(-7.99999999999999,0.,0.));
#8939=CARTESIAN_POINT('Origin',(8.,0.,0.));
#8940=CARTESIAN_POINT('Origin',(10.,0.,0.));
#8941=CARTESIAN_POINT('',(10.,-6.,6.));
#8942=CARTESIAN_POINT('',(10.,6.,6.));
#8943=CARTESIAN_POINT('',(10.,-6.,6.));
#8944=CARTESIAN_POINT('',(10.,6.,-6.));
#8945=CARTESIAN_POINT('',(10.,6.,6.));
#8946=CARTESIAN_POINT('',(10.,-6.,-6.));
#8947=CARTESIAN_POINT('',(10.,6.,-6.));
#8948=CARTESIAN_POINT('',(10.,-6.,-6.));
#8949=CARTESIAN_POINT('Origin',(-10.,0.,0.));
#8950=CARTESIAN_POINT('',(-10.,6.,6.));
#8951=CARTESIAN_POINT('',(-10.,6.,-6.));
#8952=CARTESIAN_POINT('',(-10.,6.,6.));
#8953=CARTESIAN_POINT('',(-10.,-6.,6.));
#8954=CARTESIAN_POINT('',(-10.,-6.,6.));
#8955=CARTESIAN_POINT('',(-10.,-6.,-6.));
#8956=CARTESIAN_POINT('',(-10.,-6.,-6.));
#8957=CARTESIAN_POINT('',(-10.,6.,-6.));
#8958=CARTESIAN_POINT('Origin',(10.,6.,6.));
#8959=CARTESIAN_POINT('',(10.,6.,6.));
#8960=CARTESIAN_POINT('',(10.,-6.,6.));
#8961=CARTESIAN_POINT('Origin',(10.,-6.,-6.));
#8962=CARTESIAN_POINT('',(10.,-6.,-6.));
#8963=CARTESIAN_POINT('Origin',(10.,6.,-6.));
#8964=CARTESIAN_POINT('',(10.,6.,-6.));
#8965=CARTESIAN_POINT('Origin',(10.,6.,-6.));
#8966=CARTESIAN_POINT('Origin',(8.,0.,0.));
#8967=CARTESIAN_POINT('Origin',(-8.,0.,0.));
#8968=CARTESIAN_POINT('Origin',(-8.,0.,0.));
#8969=CARTESIAN_POINT('Origin',(8.,0.,0.));
#8970=CARTESIAN_POINT('Origin',(8.,0.,0.));
#8971=CARTESIAN_POINT('Origin',(8.,0.,0.));
#8972=CARTESIAN_POINT('Origin',(-8.,0.,0.));
#8973=CARTESIAN_POINT('Origin',(-8.,0.,0.));
#8974=CARTESIAN_POINT('Ctrl Pts',(6.0682882506545,-70.5788750615323,8.18308311042592));
#8975=CARTESIAN_POINT('Ctrl Pts',(5.9459930489019,-70.7379930471477,6.));
#8976=CARTESIAN_POINT('Ctrl Pts',(7.2819459007854,-68.9997880838913,6.));
#8977=CARTESIAN_POINT('Ctrl Pts',(5.85289506900496,-70.4128282844964,8.18739110257159));
#8978=CARTESIAN_POINT('Ctrl Pts',(5.73151885261032,-70.5791653100974,5.99999999999939));
#8979=CARTESIAN_POINT('Ctrl Pts',(7.02347408295405,-68.801131325923,6.));
#8980=CARTESIAN_POINT('Ctrl Pts',(5.40466236457489,-70.0955016700879,8.19569728364092));
#8981=CARTESIAN_POINT('Ctrl Pts',(5.28635953512335,-70.2763620707944,6.00000000000028));
#8982=CARTESIAN_POINT('Ctrl Pts',(6.48559483742278,-68.4215002698136,6.));
#8983=CARTESIAN_POINT('Ctrl Pts',(4.46468935872559,-69.5403906874137,8.21045268554692));
#8984=CARTESIAN_POINT('Ctrl Pts',(4.35736242456404,-69.7487777423901,5.99999999999983));
#8985=CARTESIAN_POINT('Ctrl Pts',(5.35762723050994,-67.7574456427915,6.));
#8986=CARTESIAN_POINT('Ctrl Pts',(3.47443845681706,-69.108155810847,8.22218977274494));
#8987=CARTESIAN_POINT('Ctrl Pts',(3.38589325352388,-69.3410267184102,6.00000000000002));
#8988=CARTESIAN_POINT('Ctrl Pts',(4.16932614817419,-67.2404353101984,6.));
#8989=CARTESIAN_POINT('Ctrl Pts',(2.42716688477256,-68.7967926230682,8.23074835772877));
#8990=CARTESIAN_POINT('Ctrl Pts',(2.36326077208656,-69.0481924834197,6.));
#8991=CARTESIAN_POINT('Ctrl Pts',(2.91260026172825,-66.8680260601435,6.));
#8992=CARTESIAN_POINT('Ctrl Pts',(1.6218304880885,-68.6287353881328,8.23540093540621));
#8993=CARTESIAN_POINT('Ctrl Pts',(1.57815237662727,-68.8903657331695,6.));
#8994=CARTESIAN_POINT('Ctrl Pts',(1.94619658570589,-66.6670266084519,6.));
#8995=CARTESIAN_POINT('Ctrl Pts',(0.810640842823951,-68.5282345115354,8.23819625965817));
#8996=CARTESIAN_POINT('Ctrl Pts',(0.788515249238892,-68.7961066876711,6.));
#8997=CARTESIAN_POINT('Ctrl Pts',(0.972769011388829,-66.5468286047189,6.));
#8998=CARTESIAN_POINT('Ctrl Pts',(-0.0132433122964684,-68.4950325348177,
8.23912191540781));
#8999=CARTESIAN_POINT('Ctrl Pts',(-0.0128812315317467,-68.7649879925767,
6.));
#9000=CARTESIAN_POINT('Ctrl Pts',(-0.0158919747557947,-66.5071198611988,
6.));
#9001=CARTESIAN_POINT('Ctrl Pts',(-0.827108987367283,-68.5298673022841,
8.23815076810972));
#9002=CARTESIAN_POINT('Ctrl Pts',(-0.804540023139105,-68.7976373398413,
6.));
#9003=CARTESIAN_POINT('Ctrl Pts',(-0.992530784840697,-66.5487813885413,
6.));
#9004=CARTESIAN_POINT('Ctrl Pts',(-1.63242644644223,-68.63073424706,8.23534551400686));
#9005=CARTESIAN_POINT('Ctrl Pts',(-1.58848648494722,-68.8922433071613,6.));
#9006=CARTESIAN_POINT('Ctrl Pts',(-1.95891173573081,-66.6694172614361,6.));
#9007=CARTESIAN_POINT('Ctrl Pts',(-2.42769216080527,-68.7970511938874,8.23074135526182));
#9008=CARTESIAN_POINT('Ctrl Pts',(-2.36377796144039,-69.048438722032,6.));
#9009=CARTESIAN_POINT('Ctrl Pts',(-2.91323059296582,-66.8683353480222,6.));
#9010=CARTESIAN_POINT('Ctrl Pts',(-3.21763744666268,-69.0317566304427,8.22428947864325));
#9011=CARTESIAN_POINT('Ctrl Pts',(-3.13559523629935,-69.2692975136533,6.));
#9012=CARTESIAN_POINT('Ctrl Pts',(-3.86116493599712,-67.1490571952379,6.));
#9013=CARTESIAN_POINT('Ctrl Pts',(-3.97822064659548,-69.3282657416192,8.21621403377884));
#9014=CARTESIAN_POINT('Ctrl Pts',(-3.88090592793965,-69.549032366911,6.00000000000002));
#9015=CARTESIAN_POINT('Ctrl Pts',(-4.77386477590747,-67.5037162736474,6.));
#9016=CARTESIAN_POINT('Ctrl Pts',(-4.70828444236236,-69.6838200040427,8.20663923051075));
#9017=CARTESIAN_POINT('Ctrl Pts',(-4.5988151491346,-69.8854869172508,5.99999999999994));
#9018=CARTESIAN_POINT('Ctrl Pts',(-5.64994133086137,-67.9290235661228,6.));
#9019=CARTESIAN_POINT('Ctrl Pts',(-5.40786575147718,-70.0977834228121,8.19563756564667));
#9020=CARTESIAN_POINT('Ctrl Pts',(-5.28954603953759,-70.2785444703306,6.00000000000021));
#9021=CARTESIAN_POINT('Ctrl Pts',(-6.48943890167358,-68.4242300266046,6.));
#9022=CARTESIAN_POINT('Ctrl Pts',(-5.85541803997558,-70.4145999513425,8.18734468717341));
#9023=CARTESIAN_POINT('Ctrl Pts',(-5.73401743225063,-70.5808509979729,5.99999999999954));
#9024=CARTESIAN_POINT('Ctrl Pts',(-7.02650164818409,-68.8032508361093,6.));
#9025=CARTESIAN_POINT('Ctrl Pts',(-6.07230111177522,-70.5819701972286,8.18300281304048));
#9026=CARTESIAN_POINT('Ctrl Pts',(-5.94998411612338,-70.7409501459778,6.));
#9027=CARTESIAN_POINT('Ctrl Pts',(-7.28676133413026,-69.0034910751822,6.));
#9028=CARTESIAN_POINT('Ctrl Pts',(-6.06803252706027,-70.5786779305751,-8.18308822489702));
#9029=CARTESIAN_POINT('Ctrl Pts',(-5.94573871849779,-70.7378047103369,-6.));
#9030=CARTESIAN_POINT('Ctrl Pts',(-7.28163903247233,-68.9995522383246,-6.));
#9031=CARTESIAN_POINT('Ctrl Pts',(-5.85347731350505,-70.4132881638106,-8.1873791998786));
#9032=CARTESIAN_POINT('Ctrl Pts',(-5.73210035380063,-70.579606412197,-5.99999999999983));
#9033=CARTESIAN_POINT('Ctrl Pts',(-7.02417277625494,-68.8016815272326,-6.));
#9034=CARTESIAN_POINT('Ctrl Pts',(-5.4111283081438,-70.0998002542412,-8.19558414953762));
#9035=CARTESIAN_POINT('Ctrl Pts',(-5.29276551111711,-70.2804580835622,-6.00000000000008));
#9036=CARTESIAN_POINT('Ctrl Pts',(-6.49335396974988,-68.4266427135835,-6.));
#9037=CARTESIAN_POINT('Ctrl Pts',(-4.70118346556066,-69.6796411462325,-8.20675036532539));
#9038=CARTESIAN_POINT('Ctrl Pts',(-4.59178484404709,-69.8815086667827,-5.99999999999998));
#9039=CARTESIAN_POINT('Ctrl Pts',(-5.64142015867887,-67.9240245960956,-6.));
#9040=CARTESIAN_POINT('Ctrl Pts',(-3.96654205942963,-69.3231600030763,-8.21635249184322));
#9041=CARTESIAN_POINT('Ctrl Pts',(-3.86944503708174,-69.5442114415875,-6.));
#9042=CARTESIAN_POINT('Ctrl Pts',(-4.75985047131393,-67.4976090926177,-6.));
#9043=CARTESIAN_POINT('Ctrl Pts',(-3.20951506433543,-69.0293095986277,-8.22435673696605));
#9044=CARTESIAN_POINT('Ctrl Pts',(-3.12767187365864,-69.2669987740208,-6.));
#9045=CARTESIAN_POINT('Ctrl Pts',(-3.85141807720296,-67.1461303958146,-6.));
#9046=CARTESIAN_POINT('Ctrl Pts',(-2.43078328288814,-68.7978816199521,-8.23071847511551));
#9047=CARTESIAN_POINT('Ctrl Pts',(-2.36679776159459,-69.0492202784216,-6.));
#9048=CARTESIAN_POINT('Ctrl Pts',(-2.91693993946566,-66.8693285762601,-6.));
#9049=CARTESIAN_POINT('Ctrl Pts',(-1.62586716451067,-68.6292738987564,-8.23538592349982));
#9050=CARTESIAN_POINT('Ctrl Pts',(-1.58208021199484,-68.8908695978791,-6.));
#9051=CARTESIAN_POINT('Ctrl Pts',(-1.95104059741283,-66.6676706545943,-6.));
#9052=CARTESIAN_POINT('Ctrl Pts',(-0.811246104747758,-68.528376006915,-8.23819232856168));
#9053=CARTESIAN_POINT('Ctrl Pts',(-0.789104003287774,-68.7962395994468,
-6.));
#9054=CARTESIAN_POINT('Ctrl Pts',(-0.973495325697306,-66.5469978325812,
-6.));
#9055=CARTESIAN_POINT('Ctrl Pts',(0.00694046074342192,-68.4949754898681,
-8.23912350096698));
#9056=CARTESIAN_POINT('Ctrl Pts',(0.0067491433536535,-68.7649343963049,
-6.));
#9057=CARTESIAN_POINT('Ctrl Pts',(0.00832855289212235,-66.5070516358273,
-6.));
#9058=CARTESIAN_POINT('Ctrl Pts',(0.830469565512463,-68.5299319685166,-8.23814897045333));
#9059=CARTESIAN_POINT('Ctrl Pts',(0.80780778884349,-68.7976980585048,-6.));
#9060=CARTESIAN_POINT('Ctrl Pts',(0.996563478614889,-66.5488587288769,-6.));
#9061=CARTESIAN_POINT('Ctrl Pts',(1.63747646581493,-68.6315544877087,-8.23532268183347));
#9062=CARTESIAN_POINT('Ctrl Pts',(1.59340092659167,-68.8930115216497,-6.));
#9063=CARTESIAN_POINT('Ctrl Pts',(1.96497175897817,-66.6703982568214,-6.));
#9064=CARTESIAN_POINT('Ctrl Pts',(2.43210940714635,-68.7983855401701,-8.23070470254197));
#9065=CARTESIAN_POINT('Ctrl Pts',(2.36810398473332,-69.0496973102161,-6.));
#9066=CARTESIAN_POINT('Ctrl Pts',(2.91853128857469,-66.8699313126498,-6.));
#9067=CARTESIAN_POINT('Ctrl Pts',(3.21272958292764,-69.0301041506723,-8.22433471552509));
#9068=CARTESIAN_POINT('Ctrl Pts',(3.13079385880829,-69.2677406291319,-6.00000000000001));
#9069=CARTESIAN_POINT('Ctrl Pts',(3.85527549951665,-67.1470806885609,-6.));
#9070=CARTESIAN_POINT('Ctrl Pts',(3.98172154951034,-69.3295276483392,-8.21617950273701));
#9071=CARTESIAN_POINT('Ctrl Pts',(3.88432273738468,-69.5502163162855,-5.99999999999995));
#9072=CARTESIAN_POINT('Ctrl Pts',(4.77806585939939,-67.5052256260813,-6.));
#9073=CARTESIAN_POINT('Ctrl Pts',(4.95801912054651,-69.8059991662796,-8.20334997367537));
#9074=CARTESIAN_POINT('Ctrl Pts',(4.84354578298823,-70.0007101356207,-6.00000000000025));
#9075=CARTESIAN_POINT('Ctrl Pts',(5.94962294472498,-68.0751721643964,-6.));
#9076=CARTESIAN_POINT('Ctrl Pts',(5.64014398919804,-70.2485011895088,-8.19165365412494));
#9077=CARTESIAN_POINT('Ctrl Pts',(5.51914430293978,-70.4215908515748,-5.99999999999891));
#9078=CARTESIAN_POINT('Ctrl Pts',(6.76817278673088,-68.6045318062231,-6.));
#9079=CARTESIAN_POINT('Ctrl Pts',(6.07195815035803,-70.5817055432315,-8.18300967865433));
#9080=CARTESIAN_POINT('Ctrl Pts',(5.94964301231408,-70.740697292135,-6.));
#9081=CARTESIAN_POINT('Ctrl Pts',(7.28634978042964,-69.0031744455552,-6.));
#9082=CARTESIAN_POINT('Ctrl Pts',(6.06801845291636,8.1830885063712,70.578667081549));
#9083=CARTESIAN_POINT('Ctrl Pts',(5.94572472104539,6.00000000000025,70.7377943453019));
#9084=CARTESIAN_POINT('Ctrl Pts',(7.28162214349963,6.00000000000024,68.9995392586552));
#9085=CARTESIAN_POINT('Ctrl Pts',(5.85350545654079,8.18737862287716,70.4133104642334));
#9086=CARTESIAN_POINT('Ctrl Pts',(5.73212846769281,5.99999999999972,70.579627806427));
#9087=CARTESIAN_POINT('Ctrl Pts',(7.02420654789107,6.00000000000024,68.8017082075856));
#9088=CARTESIAN_POINT('Ctrl Pts',(5.41142083747605,8.19557825641887,70.1000263112598));
#9089=CARTESIAN_POINT('Ctrl Pts',(5.29305834816035,6.0000000000005,70.280674868654));
#9090=CARTESIAN_POINT('Ctrl Pts',(6.49370500495172,6.00000000000024,68.4269131601669));
#9091=CARTESIAN_POINT('Ctrl Pts',(4.70226077585541,8.2067352102742,69.680206595972));
#9092=CARTESIAN_POINT('Ctrl Pts',(4.59284510950782,6.00000000000018,69.8820441142854));
#9093=CARTESIAN_POINT('Ctrl Pts',(5.64271293103173,6.00000000000024,67.9247009918506));
#9094=CARTESIAN_POINT('Ctrl Pts',(3.96640109231569,8.21635488943785,69.3230697140021));
#9095=CARTESIAN_POINT('Ctrl Pts',(3.86930402127679,6.00000000000027,69.5441249357653));
#9096=CARTESIAN_POINT('Ctrl Pts',(4.75968131077742,6.00000000000024,67.497501083266));
#9097=CARTESIAN_POINT('Ctrl Pts',(3.20933677074826,8.22435834530184,69.0292514433744));
#9098=CARTESIAN_POINT('Ctrl Pts',(3.12749804869432,6.00000000000024,69.2669443838855));
#9099=CARTESIAN_POINT('Ctrl Pts',(3.85120412489829,6.00000000000023,67.1460608406989));
#9100=CARTESIAN_POINT('Ctrl Pts',(2.43079492950821,8.23071752336813,68.7979164367695));
#9101=CARTESIAN_POINT('Ctrl Pts',(2.36681062468134,6.00000000000025,69.0492532338038));
#9102=CARTESIAN_POINT('Ctrl Pts',(2.91695391540976,6.00000000000023,66.8693702204437));
#9103=CARTESIAN_POINT('Ctrl Pts',(1.62719099386776,8.23537981519032,68.6294940882333));
#9104=CARTESIAN_POINT('Ctrl Pts',(1.5833700332159,6.00000000000025,68.8910763437912));
#9105=CARTESIAN_POINT('Ctrl Pts',(1.95262919264134,6.00000000000024,66.6679340024137));
#9106=CARTESIAN_POINT('Ctrl Pts',(0.811476579102376,8.23819216142386,68.5283818247723));
#9107=CARTESIAN_POINT('Ctrl Pts',(0.789327567123226,6.00000000000025,68.7962449283322));
#9108=CARTESIAN_POINT('Ctrl Pts',(0.973771894922848,6.00000000000023,66.5470047895178));
#9109=CARTESIAN_POINT('Ctrl Pts',(-0.00607573808073577,8.23912316054545,
68.494987768917));
#9110=CARTESIAN_POINT('Ctrl Pts',(-0.00590784164394143,6.00000000000025,
68.764945955377));
#9111=CARTESIAN_POINT('Ctrl Pts',(-0.007290885696897,6.00000000000023,66.5070663216835));
#9112=CARTESIAN_POINT('Ctrl Pts',(-0.830079220669207,8.23815058533074,68.5298739460195));
#9113=CARTESIAN_POINT('Ctrl Pts',(-0.807427697439417,6.00000000000025,68.7976436237591));
#9114=CARTESIAN_POINT('Ctrl Pts',(-0.996095064802989,6.00000000000023,66.5487893348009));
#9115=CARTESIAN_POINT('Ctrl Pts',(-1.63783143137718,8.23532139951924,68.6316004941713));
#9116=CARTESIAN_POINT('Ctrl Pts',(-1.59374595912617,6.00000000000025,68.8930545679141));
#9117=CARTESIAN_POINT('Ctrl Pts',(-1.96539771765284,6.00000000000024,66.670453279486));
#9118=CARTESIAN_POINT('Ctrl Pts',(-2.4324940845882,8.23070164698601,68.7984964593138));
#9119=CARTESIAN_POINT('Ctrl Pts',(-2.36848014491559,6.00000000000025,69.0498017139277));
#9120=CARTESIAN_POINT('Ctrl Pts',(-2.91899290150501,6.00000000000023,66.8700639772304));
#9121=CARTESIAN_POINT('Ctrl Pts',(-3.21237058587918,8.22433751057345,69.0300029226234));
#9122=CARTESIAN_POINT('Ctrl Pts',(-3.13044430354236,6.00000000000025,69.2676458481511));
#9123=CARTESIAN_POINT('Ctrl Pts',(-3.85484470305812,6.00000000000024,67.1469596163795));
#9124=CARTESIAN_POINT('Ctrl Pts',(-3.98123403834483,8.21618579285133,69.3292945527418));
#9125=CARTESIAN_POINT('Ctrl Pts',(-3.88384257406888,6.00000000000025,69.5499954728079));
#9126=CARTESIAN_POINT('Ctrl Pts',(-4.77748084600222,6.00000000000024,67.5049468043074));
#9127=CARTESIAN_POINT('Ctrl Pts',(-4.9587261495966,8.20334062563248,69.8063458318945));
#9128=CARTESIAN_POINT('Ctrl Pts',(-4.84423794709568,6.00000000000025,70.001036400311));
#9129=CARTESIAN_POINT('Ctrl Pts',(-5.95047137957739,6.00000000000024,68.0755868366564));
#9130=CARTESIAN_POINT('Ctrl Pts',(-5.64048203786072,8.19164677753803,70.2487667358696));
#9131=CARTESIAN_POINT('Ctrl Pts',(-5.51948258067411,6.00000000000029,70.4218460646259));
#9132=CARTESIAN_POINT('Ctrl Pts',(-6.76857844516023,6.00000000000024,68.6048495059982));
#9133=CARTESIAN_POINT('Ctrl Pts',(-6.07190402898392,8.1830107620393,70.5816637813997));
#9134=CARTESIAN_POINT('Ctrl Pts',(-5.94958918416741,6.00000000000025,70.7406573923915));
#9135=CARTESIAN_POINT('Ctrl Pts',(-7.2862848347807,6.00000000000024,69.0031244820821));
#9136=CARTESIAN_POINT('Ctrl Pts',(-6.06834088416797,-8.18308205771751,70.5789156370285));
#9137=CARTESIAN_POINT('Ctrl Pts',(-5.94604539573102,-5.99999999999975,70.7380318125804));
#9138=CARTESIAN_POINT('Ctrl Pts',(-7.28200906100156,-5.99999999999976,68.9998366280225));
#9139=CARTESIAN_POINT('Ctrl Pts',(-5.85277105864604,-8.18739363605577,70.4127304061065));
#9140=CARTESIAN_POINT('Ctrl Pts',(-5.73139500673848,-6.00000000000109,70.5790714320876));
#9141=CARTESIAN_POINT('Ctrl Pts',(-7.02332527052808,-5.99999999999976,68.8010142238958));
#9142=CARTESIAN_POINT('Ctrl Pts',(-5.40389248678053,-8.1957102200564,70.0950123273115));
#9143=CARTESIAN_POINT('Ctrl Pts',(-5.28559866593569,-5.99999999999914,70.2758971643673));
#9144=CARTESIAN_POINT('Ctrl Pts',(-6.48467098406741,-5.99999999999976,68.4209148757263));
#9145=CARTESIAN_POINT('Ctrl Pts',(-4.46552260677635,-8.21043868494446,69.5409186810962));
#9146=CARTESIAN_POINT('Ctrl Pts',(-4.35819209250992,-6.00000000000011,69.7492824480618));
#9147=CARTESIAN_POINT('Ctrl Pts',(-5.3586271281721,-5.99999999999976,67.7580772654495));
#9148=CARTESIAN_POINT('Ctrl Pts',(-3.4753489624829,-8.22218339603287,69.1083854232455));
#9149=CARTESIAN_POINT('Ctrl Pts',(-3.38677700455703,-5.9999999999997,69.3412405452436));
#9150=CARTESIAN_POINT('Ctrl Pts',(-4.170418754973,-5.99999999999977,67.2407099265433));
#9151=CARTESIAN_POINT('Ctrl Pts',(-2.42624705360006,-8.23075476367214,68.7965605885707));
#9152=CARTESIAN_POINT('Ctrl Pts',(-2.36236305382706,-5.99999999999976,69.0479744163574));
#9153=CARTESIAN_POINT('Ctrl Pts',(-2.91149646432129,-5.99999999999977,66.8677485388432));
#9154=CARTESIAN_POINT('Ctrl Pts',(-1.62204779908062,-8.23539943445322,68.6287897669284));
#9155=CARTESIAN_POINT('Ctrl Pts',(-1.57836506118308,-5.99999999999975,68.8904169809383));
#9156=CARTESIAN_POINT('Ctrl Pts',(-1.94645735889641,-5.99999999999977,66.6670916474468));
#9157=CARTESIAN_POINT('Ctrl Pts',(-0.810375770559074,-8.23819731057242,
68.5281966361225));
#9158=CARTESIAN_POINT('Ctrl Pts',(-0.78825681439635,-5.99999999999975,68.796071073066));
#9159=CARTESIAN_POINT('Ctrl Pts',(-0.972450924670978,-5.99999999999977,
66.5467833055616));
#9160=CARTESIAN_POINT('Ctrl Pts',(0.0133055089948572,-8.23912127759622,
68.4950554619354));
#9161=CARTESIAN_POINT('Ctrl Pts',(0.0129415792074661,-5.99999999999975,
68.7650095211385));
#9162=CARTESIAN_POINT('Ctrl Pts',(0.0159666107938615,-5.99999999999977,
66.5071472817672));
#9163=CARTESIAN_POINT('Ctrl Pts',(0.826267631217788,-8.23815227908787,68.529813087084));
#9164=CARTESIAN_POINT('Ctrl Pts',(0.803721811298467,-5.99999999999975,68.7975865283896));
#9165=CARTESIAN_POINT('Ctrl Pts',(0.991521157461304,-5.99999999999977,66.5487165483907));
#9166=CARTESIAN_POINT('Ctrl Pts',(1.63154625951178,-8.23534985135178,68.6305780621835));
#9167=CARTESIAN_POINT('Ctrl Pts',(1.58762892121974,-5.99999999999975,68.8920967742542));
#9168=CARTESIAN_POINT('Ctrl Pts',(1.95785551141427,-5.99999999999977,66.6692304644635));
#9169=CARTESIAN_POINT('Ctrl Pts',(2.42740394362686,-8.23074402945943,68.7969536012691));
#9170=CARTESIAN_POINT('Ctrl Pts',(2.36349505098862,-5.99999999999975,69.0483465087462));
#9171=CARTESIAN_POINT('Ctrl Pts',(2.91288473235175,-5.99999999999976,66.8682186195194));
#9172=CARTESIAN_POINT('Ctrl Pts',(3.21782649539177,-8.22428729467809,69.0318370973241));
#9173=CARTESIAN_POINT('Ctrl Pts',(3.13578143863181,-5.99999999999976,69.2693737863226));
#9174=CARTESIAN_POINT('Ctrl Pts',(3.86139179447194,-5.99999999999977,67.1491534445295));
#9175=CARTESIAN_POINT('Ctrl Pts',(3.97730474384737,-8.21622429420431,69.3278879313072));
#9176=CARTESIAN_POINT('Ctrl Pts',(3.880008753726,-5.99999999999972,69.5486760172004));
#9177=CARTESIAN_POINT('Ctrl Pts',(4.77276569261006,-5.99999999999977,67.5032643626668));
#9178=CARTESIAN_POINT('Ctrl Pts',(4.70742733158002,-8.20665165144787,69.6833563763738));
#9179=CARTESIAN_POINT('Ctrl Pts',(4.59797063943759,-5.99999999999986,69.8850477806615));
#9180=CARTESIAN_POINT('Ctrl Pts',(5.64891279792138,-5.99999999999976,67.9284689696251));
#9181=CARTESIAN_POINT('Ctrl Pts',(5.40725025962937,-8.19564900701384,70.0973460631149));
#9182=CARTESIAN_POINT('Ctrl Pts',(5.28893319868001,-5.99999999999934,70.2781260183458));
#9183=CARTESIAN_POINT('Ctrl Pts',(6.48870031146062,-5.99999999999976,68.4237067935522));
#9184=CARTESIAN_POINT('Ctrl Pts',(5.85561464211331,-8.18734066811789,70.4147552346278));
#9185=CARTESIAN_POINT('Ctrl Pts',(5.73421377853935,-6.00000000000062,70.5809999378274));
#9186=CARTESIAN_POINT('Ctrl Pts',(7.02673757073987,-5.99999999999976,68.8034366175773));
#9187=CARTESIAN_POINT('Ctrl Pts',(6.07221930260315,-8.183004450797,70.5819070651678));
#9188=CARTESIAN_POINT('Ctrl Pts',(5.94990274997528,-5.99999999999975,70.7408898287435));
#9189=CARTESIAN_POINT('Ctrl Pts',(7.28666316312378,-5.99999999999976,69.0034155445595));
#9190=CARTESIAN_POINT('Ctrl Pts',(6.06875473483189,-8.18309759645187,-70.5792319349097));
#9191=CARTESIAN_POINT('Ctrl Pts',(5.94643964085432,-6.00000000000025,-70.7383565071141));
#9192=CARTESIAN_POINT('Ctrl Pts',(7.28250408242006,-6.00000000000024,-69.0002171181955));
#9193=CARTESIAN_POINT('Ctrl Pts',(5.85178703948071,-8.18743757171489,-70.4119510234682));
#9194=CARTESIAN_POINT('Ctrl Pts',(5.73039546650288,-5.99999999999948,-70.5783470003785));
#9195=CARTESIAN_POINT('Ctrl Pts',(7.02214286219319,-6.00000000000024,-68.8000839347804));
#9196=CARTESIAN_POINT('Ctrl Pts',(5.40413875921895,-8.19572501730264,-70.095371489302));
#9197=CARTESIAN_POINT('Ctrl Pts',(5.28584267076014,-6.00000000000061,-70.2762746863069));
#9198=CARTESIAN_POINT('Ctrl Pts',(6.48496496950678,-6.00000000000024,-68.4213469913216));
#9199=CARTESIAN_POINT('Ctrl Pts',(4.70453541541043,-8.20671705513184,-69.6818030748008));
#9200=CARTESIAN_POINT('Ctrl Pts',(4.59510783781567,-6.00000000000016,-69.8836011976203));
#9201=CARTESIAN_POINT('Ctrl Pts',(5.64544107697617,-6.00000000000024,-67.9266134977138));
#9202=CARTESIAN_POINT('Ctrl Pts',(3.97447865414692,-8.21628193502219,-69.3266412584454));
#9203=CARTESIAN_POINT('Ctrl Pts',(3.87722246833469,-6.00000000000028,-69.5475251536455));
#9204=CARTESIAN_POINT('Ctrl Pts',(4.76937312491094,-6.00000000000024,-67.5017760124435));
#9205=CARTESIAN_POINT('Ctrl Pts',(3.21437312354095,-8.22434380390216,-69.0306454426741));
#9206=CARTESIAN_POINT('Ctrl Pts',(3.13239258384128,-6.00000000000024,-69.2682791211047));
#9207=CARTESIAN_POINT('Ctrl Pts',(3.85724668850695,-6.00000000000024,-67.1477311850147));
#9208=CARTESIAN_POINT('Ctrl Pts',(2.42376825729524,-8.23079411637547,-68.7960041651443));
#9209=CARTESIAN_POINT('Ctrl Pts',(2.35993781294462,-6.00000000000025,-69.0474823212491));
#9210=CARTESIAN_POINT('Ctrl Pts',(2.9085210851309,-6.00000000000024,-66.8670862868854));
#9211=CARTESIAN_POINT('Ctrl Pts',(1.62381972536018,-8.2354160205023,-68.6290551598252));
#9212=CARTESIAN_POINT('Ctrl Pts',(1.58008663699865,-6.00000000000025,-68.8906963954579));
#9213=CARTESIAN_POINT('Ctrl Pts',(1.94858310686874,-6.00000000000023,-66.6674124238467));
#9214=CARTESIAN_POINT('Ctrl Pts',(0.806804782644178,-8.238230881506,-68.527846491126));
#9215=CARTESIAN_POINT('Ctrl Pts',(0.784779198305824,-6.00000000000025,-68.795769877695));
#9216=CARTESIAN_POINT('Ctrl Pts',(0.96816545556796,-6.00000000000023,-66.5463679508953));
#9217=CARTESIAN_POINT('Ctrl Pts',(-0.283444643618167,-8.23943970404702,
-68.4845142474358));
#9218=CARTESIAN_POINT('Ctrl Pts',(-0.275801169709708,-6.00000000000025,
-68.7551714931309));
#9219=CARTESIAN_POINT('Ctrl Pts',(-0.340133473956596,-6.00000000000023,
-66.4945438531381));
#9220=CARTESIAN_POINT('Ctrl Pts',(-1.62860970393417,-8.23633611996313,-68.595645744352));
#9221=CARTESIAN_POINT('Ctrl Pts',(-1.58330020161186,-6.00000000000027,-68.8591514885485));
#9222=CARTESIAN_POINT('Ctrl Pts',(-1.9543310609976,-6.00000000000023,-66.6274531349024));
#9223=CARTESIAN_POINT('Ctrl Pts',(-3.2312143093488,-8.22512639339453,-69.0008899721718));
#9224=CARTESIAN_POINT('Ctrl Pts',(-3.14620792364501,-6.00000000000017,-69.2394478237357));
#9225=CARTESIAN_POINT('Ctrl Pts',(-3.87745607258566,-6.00000000000024,-67.1121341857481));
#9226=CARTESIAN_POINT('Ctrl Pts',(-4.46858440416536,-8.21042143575268,-69.5424343805895));
#9227=CARTESIAN_POINT('Ctrl Pts',(-4.36118635957745,-6.00000000000049,-69.7507353701984));
#9228=CARTESIAN_POINT('Ctrl Pts',(-5.36229989129301,-6.00000000000024,-67.759892952126));
#9229=CARTESIAN_POINT('Ctrl Pts',(-5.4083833220806,-8.19565805801412,-70.0978905482687));
#9230=CARTESIAN_POINT('Ctrl Pts',(-5.29002494401106,-5.99999999999985,-70.2786591175671));
#9231=CARTESIAN_POINT('Ctrl Pts',(-6.49005844414082,-6.00000000000024,-68.4243604294078));
#9232=CARTESIAN_POINT('Ctrl Pts',(-5.85649506183581,-8.18734650418252,-70.4154478176525));
#9233=CARTESIAN_POINT('Ctrl Pts',(-5.73507620737369,-6.00000000000114,-70.5816873084557));
#9234=CARTESIAN_POINT('Ctrl Pts',(-7.0277924885399,-6.00000000000024,-68.8042673910917));
#9235=CARTESIAN_POINT('Ctrl Pts',(-6.07185145156228,-8.18303563075614,-70.5816204501341));
#9236=CARTESIAN_POINT('Ctrl Pts',(-5.94951953188762,-6.00000000000025,-70.7406384910899));
#9237=CARTESIAN_POINT('Ctrl Pts',(-7.28622014224927,-6.00000000000024,-69.0030747140361));
#9238=CARTESIAN_POINT('Ctrl Pts',(-6.06801871741568,8.18308850108089,-70.5786672854375));
#9239=CARTESIAN_POINT('Ctrl Pts',(-5.94572498410341,5.99999999999975,-70.7377945400946));
#9240=CARTESIAN_POINT('Ctrl Pts',(-7.28162246089882,5.99999999999976,-68.9995395025853));
#9241=CARTESIAN_POINT('Ctrl Pts',(-5.6389103743372,8.19167038155535,-70.2478905485423));
#9242=CARTESIAN_POINT('Ctrl Pts',(-5.51794464646817,6.00000000000053,-70.4210261561648));
#9243=CARTESIAN_POINT('Ctrl Pts',(-6.76669244916325,5.99999999999976,-68.6038014271042));
#9244=CARTESIAN_POINT('Ctrl Pts',(-4.95704234660675,8.20338648207493,-69.8045805431969));
#9245=CARTESIAN_POINT('Ctrl Pts',(-4.84250783046514,5.99999999999957,-69.9993321538736));
#9246=CARTESIAN_POINT('Ctrl Pts',(-5.94845081593742,5.99999999999976,-68.0734748718918));
#9247=CARTESIAN_POINT('Ctrl Pts',(-3.96744158691016,8.21634812748047,-69.3233047664328));
#9248=CARTESIAN_POINT('Ctrl Pts',(-3.87030741903311,5.99999999999978,-69.5443375003731));
#9249=CARTESIAN_POINT('Ctrl Pts',(-4.76092990429044,5.99999999999976,-67.4977821572228));
#9250=CARTESIAN_POINT('Ctrl Pts',(-3.20874982183398,8.22436433780971,-69.0290350135615));
#9251=CARTESIAN_POINT('Ctrl Pts',(-3.12692407346289,5.99999999999974,-69.2667420899));
#9252=CARTESIAN_POINT('Ctrl Pts',(-3.85049978620124,5.99999999999977,-67.1458019863229));
#9253=CARTESIAN_POINT('Ctrl Pts',(-2.43024294402271,8.23071770241596,-68.7979113655376));
#9254=CARTESIAN_POINT('Ctrl Pts',(-2.36627888415488,5.99999999999975,-69.0492494521875));
#9255=CARTESIAN_POINT('Ctrl Pts',(-2.91629153282712,5.99999999999976,-66.8693641637389));
#9256=CARTESIAN_POINT('Ctrl Pts',(-1.63363652776448,8.23534766361698,-68.6306536433433));
#9257=CARTESIAN_POINT('Ctrl Pts',(-1.5896523597654,5.99999999999975,-68.8921654789989));
#9258=CARTESIAN_POINT('Ctrl Pts',(-1.96036383331742,5.99999999999977,-66.669320840075));
#9259=CARTESIAN_POINT('Ctrl Pts',(-0.815211414748784,8.23818669105861,-68.5285770148599));
#9260=CARTESIAN_POINT('Ctrl Pts',(-0.792958661983601,5.99999999999975,-68.7964271193057));
#9261=CARTESIAN_POINT('Ctrl Pts',(-0.978253697698524,5.99999999999977,-66.5472382258622));
#9262=CARTESIAN_POINT('Ctrl Pts',(0.00264516296727683,8.23912024758092,
-68.495093664448));
#9263=CARTESIAN_POINT('Ctrl Pts',(0.00257169497954889,5.99999999999975,
-68.7650461932855));
#9264=CARTESIAN_POINT('Ctrl Pts',(0.00317419556070009,5.99999999999977,
-66.5071929785566));
#9265=CARTESIAN_POINT('Ctrl Pts',(0.82368949116962,8.23816805427952,-68.5292427295882));
#9266=CARTESIAN_POINT('Ctrl Pts',(0.801208987662387,5.99999999999975,-68.797049035209));
#9267=CARTESIAN_POINT('Ctrl Pts',(0.988427389403655,5.99999999999977,-66.5480343879385));
#9268=CARTESIAN_POINT('Ctrl Pts',(1.91030037741018,8.23437068737471,-68.6658024039292));
#9269=CARTESIAN_POINT('Ctrl Pts',(1.85869062009036,5.99999999999975,-68.9251108313631));
#9270=CARTESIAN_POINT('Ctrl Pts',(2.29236045289163,5.99999999999977,-66.7113585312388));
#9271=CARTESIAN_POINT('Ctrl Pts',(2.9578869124087,8.22702280389032,-68.9314459585039));
#9272=CARTESIAN_POINT('Ctrl Pts',(2.88034732575977,5.99999999999977,-69.1744069005992));
#9273=CARTESIAN_POINT('Ctrl Pts',(3.54946429489408,5.99999999999977,-67.0290743581477));
#9274=CARTESIAN_POINT('Ctrl Pts',(3.9746715687375,8.21626478748155,-69.3263736287728));
#9275=CARTESIAN_POINT('Ctrl Pts',(3.87739899030771,5.99999999999972,-69.5472323185878));
#9276=CARTESIAN_POINT('Ctrl Pts',(4.76960588247878,5.99999999999976,-67.5014529227093));
#9277=CARTESIAN_POINT('Ctrl Pts',(4.9619552371481,8.2033051832732,-69.8076440049128));
#9278=CARTESIAN_POINT('Ctrl Pts',(4.84737353210574,5.99999999999993,-70.0022474209937));
#9279=CARTESIAN_POINT('Ctrl Pts',(5.95434628461138,5.99999999999976,-68.0771395833567));
#9280=CARTESIAN_POINT('Ctrl Pts',(5.64195423199013,8.19161683866198,-70.249922819652));
#9281=CARTESIAN_POINT('Ctrl Pts',(5.52095572201563,5.99999999999897,-70.4229571273111));
#9282=CARTESIAN_POINT('Ctrl Pts',(6.77034507823848,5.99999999999976,-68.606232644865));
#9283=CARTESIAN_POINT('Ctrl Pts',(6.07167146824097,8.18301541721047,-70.5814843365868));
#9284=CARTESIAN_POINT('Ctrl Pts',(5.94935788369522,5.99999999999975,-70.7404859488671));
#9285=CARTESIAN_POINT('Ctrl Pts',(7.28600576188916,5.99999999999976,-69.0029097959542));
#9286=CARTESIAN_POINT('Ctrl Pts',(6.06845316111809,70.5790021938727,-8.18307981205452));
#9287=CARTESIAN_POINT('Ctrl Pts',(5.9461570612046,70.7381145081864,-6.));
#9288=CARTESIAN_POINT('Ctrl Pts',(7.28214379334171,68.9999401837949,-6.));
#9289=CARTESIAN_POINT('Ctrl Pts',(5.85250470825994,70.412520204687,-8.18739907696574));
#9290=CARTESIAN_POINT('Ctrl Pts',(5.73112901121905,70.5788698227219,-5.99999999999878));
#9291=CARTESIAN_POINT('Ctrl Pts',(7.02300565008836,68.8007627382557,-6.));
#9292=CARTESIAN_POINT('Ctrl Pts',(5.4030400778454,70.094529204984,-8.19572312550303));
#9293=CARTESIAN_POINT('Ctrl Pts',(5.2847582859253,70.2754413258182,-6.00000000000057));
#9294=CARTESIAN_POINT('Ctrl Pts',(6.4836480933326,68.420336950426,-6.));
#9295=CARTESIAN_POINT('Ctrl Pts',(4.70138175653205,69.6800775652252,-8.20673937879446));
#9296=CARTESIAN_POINT('Ctrl Pts',(4.59201175284023,69.8819393154531,-5.99999999999985));
#9297=CARTESIAN_POINT('Ctrl Pts',(5.6416581078604,67.9245467956979,-6.));
#9298=CARTESIAN_POINT('Ctrl Pts',(3.97115974367465,69.3252465860493,-8.21629593855211));
#9299=CARTESIAN_POINT('Ctrl Pts',(3.87398144459366,69.5461824566282,-6.00000000000004));
#9300=CARTESIAN_POINT('Ctrl Pts',(4.7653916924037,67.5001049460443,-6.));
#9301=CARTESIAN_POINT('Ctrl Pts',(3.21394619993446,69.0306051709583,-8.22432109821301));
#9302=CARTESIAN_POINT('Ctrl Pts',(3.13199166924711,69.2682151205242,-5.99999999999999));
#9303=CARTESIAN_POINT('Ctrl Pts',(3.85673543992293,67.1476799730556,-6.));
#9304=CARTESIAN_POINT('Ctrl Pts',(2.42484741772666,68.7962257477066,-8.23076407364235));
#9305=CARTESIAN_POINT('Ctrl Pts',(2.36099569087951,69.04766123426,-6.));
#9306=CARTESIAN_POINT('Ctrl Pts',(2.90981690127157,66.8673480706179,-6.));
#9307=CARTESIAN_POINT('Ctrl Pts',(1.62254651618572,68.6288864435827,-8.23539674526383));
#9308=CARTESIAN_POINT('Ctrl Pts',(1.5788525519209,68.8905076108765,-6.));
#9309=CARTESIAN_POINT('Ctrl Pts',(1.94705581942297,66.6672072720232,-6.));
#9310=CARTESIAN_POINT('Ctrl Pts',(0.809578703168379,68.5281112697337,-8.23819968642438));
#9311=CARTESIAN_POINT('Ctrl Pts',(0.787480259127005,68.795990972133,-6.));
#9312=CARTESIAN_POINT('Ctrl Pts',(0.971494443802027,66.5466812084756,-6.));
#9313=CARTESIAN_POINT('Ctrl Pts',(-0.013029712981914,68.4951024671821,-8.23911996777312));
#9314=CARTESIAN_POINT('Ctrl Pts',(-0.0126728355574548,68.7650536074879,
-6.));
#9315=CARTESIAN_POINT('Ctrl Pts',(-0.0156356555782979,66.50720349905,-6.));
#9316=CARTESIAN_POINT('Ctrl Pts',(-0.82475291689116,68.5297083407777,-8.23815520081018));
#9317=CARTESIAN_POINT('Ctrl Pts',(-0.802248936456917,68.7974884178539,-6.));
#9318=CARTESIAN_POINT('Ctrl Pts',(-0.98970350026936,66.5485912747063,-6.));
#9319=CARTESIAN_POINT('Ctrl Pts',(-1.62999718711769,68.6302910463923,-8.23535781353056));
#9320=CARTESIAN_POINT('Ctrl Pts',(-1.58611884322627,68.8918272865528,-6.));
#9321=CARTESIAN_POINT('Ctrl Pts',(-1.95599662454136,66.668887192006,-6.));
#9322=CARTESIAN_POINT('Ctrl Pts',(-2.42743324168628,68.7969244893687,-8.23074480840111));
#9323=CARTESIAN_POINT('Ctrl Pts',(-2.36352138908597,69.0483185373979,-6.));
#9324=CARTESIAN_POINT('Ctrl Pts',(-2.91291989002306,66.8681837953073,-6.));
#9325=CARTESIAN_POINT('Ctrl Pts',(-3.21786438035412,69.0318882581676,-8.22428592982348));
#9326=CARTESIAN_POINT('Ctrl Pts',(-3.13582126046264,69.2694228660117,-6.));
#9327=CARTESIAN_POINT('Ctrl Pts',(-3.8614372564267,67.1492146449609,-6.));
#9328=CARTESIAN_POINT('Ctrl Pts',(-3.9757652277849,69.3272467095959,-8.21624171003073));
#9329=CARTESIAN_POINT('Ctrl Pts',(-3.87850039141612,69.548071254648,-6.));
#9330=CARTESIAN_POINT('Ctrl Pts',(-4.77091827333531,67.5024973772517,-6.));
#9331=CARTESIAN_POINT('Ctrl Pts',(-4.70599414376018,69.6825677106823,-8.2066727452182));
#9332=CARTESIAN_POINT('Ctrl Pts',(-4.59655713384728,69.8842999100366,-5.99999999999999));
#9333=CARTESIAN_POINT('Ctrl Pts',(-5.64719297253668,67.9275255515984,-6.));
#9334=CARTESIAN_POINT('Ctrl Pts',(-5.4067318828378,70.0969497733373,-8.19565931434823));
#9335=CARTESIAN_POINT('Ctrl Pts',(-5.28841438015195,70.277745403431,-6.00000000000006));
#9336=CARTESIAN_POINT('Ctrl Pts',(-6.48807825931404,68.4232326816432,-6.));
#9337=CARTESIAN_POINT('Ctrl Pts',(-5.85594494885298,70.4150161243228,-8.18733391575405));
#9338=CARTESIAN_POINT('Ctrl Pts',(-5.73454365462802,70.5812501693241,-5.99999999999987));
#9339=CARTESIAN_POINT('Ctrl Pts',(-7.02713393882033,68.80374874693,-6.));
#9340=CARTESIAN_POINT('Ctrl Pts',(-6.07208140606695,70.5818006535869,-8.18300721130884));
#9341=CARTESIAN_POINT('Ctrl Pts',(-5.94976560031573,70.7407881617334,-6.));
#9342=CARTESIAN_POINT('Ctrl Pts',(-7.28649768728034,69.003288234715,-6.));
#9343=CARTESIAN_POINT('Ctrl Pts',(-6.06800331052389,70.5786554091101,8.18308880920814));
#9344=CARTESIAN_POINT('Ctrl Pts',(-5.94570966116718,70.7377831935888,6.));
#9345=CARTESIAN_POINT('Ctrl Pts',(-7.28160397262866,68.9995252938625,6.));
#9346=CARTESIAN_POINT('Ctrl Pts',(-5.85353030598669,70.4133302716269,8.18737811067092));
#9347=CARTESIAN_POINT('Ctrl Pts',(-5.73215330255919,70.5796468161294,5.99999999999929));
#9348=CARTESIAN_POINT('Ctrl Pts',(-7.02423636720416,68.801731905345,6.));
#9349=CARTESIAN_POINT('Ctrl Pts',(-5.41162544279277,70.1002420950884,8.19557272244625));
#9350=CARTESIAN_POINT('Ctrl Pts',(-5.29326845745797,70.2808840380355,6.00000000000033));
#9351=CARTESIAN_POINT('Ctrl Pts',(-6.49395053134197,68.4271713357068,6.));
#9352=CARTESIAN_POINT('Ctrl Pts',(-4.70481487609731,69.68156698975,8.20669879137122));
#9353=CARTESIAN_POINT('Ctrl Pts',(-4.59536063894259,69.8833333373145,5.99999999999991));
#9354=CARTESIAN_POINT('Ctrl Pts',(-5.64577785131928,67.9263283153489,6.));
#9355=CARTESIAN_POINT('Ctrl Pts',(-3.96627549218016,69.3229477280658,8.21635807544407));
#9356=CARTESIAN_POINT('Ctrl Pts',(-3.8691744858435,69.5440067533137,6.00000000000002));
#9357=CARTESIAN_POINT('Ctrl Pts',(-4.75953059061551,67.4973551447454,6.));
#9358=CARTESIAN_POINT('Ctrl Pts',(-3.20911839757511,69.0291784410581,8.22436037712234));
#9359=CARTESIAN_POINT('Ctrl Pts',(-3.12728540351795,69.2668764225387,6.));
#9360=CARTESIAN_POINT('Ctrl Pts',(-3.85094207709032,67.1459735308842,6.));
#9361=CARTESIAN_POINT('Ctrl Pts',(-2.43063423668004,68.7979338632913,8.23071705603037));
#9362=CARTESIAN_POINT('Ctrl Pts',(-2.36665650885803,69.049269954688,6.));
#9363=CARTESIAN_POINT('Ctrl Pts',(-2.916761084016,66.8693910661871,6.));
#9364=CARTESIAN_POINT('Ctrl Pts',(-1.62982756087553,68.6299461600578,8.23536727988032));
#9365=CARTESIAN_POINT('Ctrl Pts',(-1.58593926432988,68.8915009519299,6.));
#9366=CARTESIAN_POINT('Ctrl Pts',(-1.95579307305065,66.6684746840155,6.));
#9367=CARTESIAN_POINT('Ctrl Pts',(-0.812141365160684,68.5283964235732,8.23819173472987));
#9368=CARTESIAN_POINT('Ctrl Pts',(-0.789973040819509,68.7962581236044,6.));
#9369=CARTESIAN_POINT('Ctrl Pts',(-0.974569638192805,66.5470222450721,6.));
#9370=CARTESIAN_POINT('Ctrl Pts',(0.00467372932650424,68.4950285445672,
8.23912206149444));
#9371=CARTESIAN_POINT('Ctrl Pts',(0.00454416602520166,68.7649851030205,
6.));
#9372=CARTESIAN_POINT('Ctrl Pts',(0.00560847519175735,66.5071150964334,
6.));
#9373=CARTESIAN_POINT('Ctrl Pts',(0.828738811659076,68.5296912309094,8.23815554792229));
#9374=CARTESIAN_POINT('Ctrl Pts',(0.80612218834234,68.797469221826,6.));
#9375=CARTESIAN_POINT('Ctrl Pts',(0.994486573991066,66.5485707839574,6.));
#9376=CARTESIAN_POINT('Ctrl Pts',(1.90845066676385,68.6658114852638,8.23437057399169));
#9377=CARTESIAN_POINT('Ctrl Pts',(1.85690343335388,68.9251227747513,6.));
#9378=CARTESIAN_POINT('Ctrl Pts',(2.29014080011569,66.7113694226116,6.));
#9379=CARTESIAN_POINT('Ctrl Pts',(2.95632883002034,68.9305419049585,8.22704718157308));
#9380=CARTESIAN_POINT('Ctrl Pts',(2.87879333312298,69.1735447167021,6.));
#9381=CARTESIAN_POINT('Ctrl Pts',(3.54759459603022,67.0279929531528,6.));
#9382=CARTESIAN_POINT('Ctrl Pts',(3.97967565233726,69.3285749611317,8.21620515776737));
#9383=CARTESIAN_POINT('Ctrl Pts',(3.88231146988333,69.5493124163549,6.00000000000001));
#9384=CARTESIAN_POINT('Ctrl Pts',(4.77561078279477,67.5040860397941,6.));
#9385=CARTESIAN_POINT('Ctrl Pts',(4.96001369761565,69.8069399276529,8.2033245920263));
#9386=CARTESIAN_POINT('Ctrl Pts',(4.84549423190842,70.0015951864197,5.99999999999992));
#9387=CARTESIAN_POINT('Ctrl Pts',(5.9520164371926,68.0762974753181,6.));
#9388=CARTESIAN_POINT('Ctrl Pts',(5.64104467416319,70.2492086476532,8.19163533365013));
#9389=CARTESIAN_POINT('Ctrl Pts',(5.52004559010036,70.4222707745883,6.00000000000035));
#9390=CARTESIAN_POINT('Ctrl Pts',(6.76925360875657,68.6053782094064,6.));
#9391=CARTESIAN_POINT('Ctrl Pts',(6.07181437220709,70.5815946005789,8.18301255673008));
#9392=CARTESIAN_POINT('Ctrl Pts',(5.94950001319883,70.7405912962541,6.));
#9393=CARTESIAN_POINT('Ctrl Pts',(7.28617724664851,69.0030417147821,6.));
#9652=UNCERTAINTY_MEASURE_WITH_UNIT(LENGTH_MEASURE(0.01),#9669,
'DISTANCE_ACCURACY_VALUE',
'Maximum model space distance between geometric entities at asserted c
onnectivities');
#9655=UNCERTAINTY_MEASURE_WITH_UNIT(LENGTH_MEASURE(0.01),#9669,
'DISTANCE_ACCURACY_VALUE',
'Maximum model space distance between geometric entities at asserted c
onnectivities');
#9665=(
GEOMETRIC_REPRESENTATION_CONTEXT(3)
GLOBAL_UNCERTAINTY_ASSIGNED_CONTEXT((#9652))
GLOBAL_UNIT_ASSIGNED_CONTEXT((#9669,#9671,#9672))
REPRESENTATION_CONTEXT('','3D')
);
#9668=(
GEOMETRIC_REPRESENTATION_CONTEXT(3)
GLOBAL_UNCERTAINTY_ASSIGNED_CONTEXT((#9655))
GLOBAL_UNIT_ASSIGNED_CONTEXT((#9669,#9671,#9672))
REPRESENTATION_CONTEXT('','3D')
);
#9669=(
LENGTH_UNIT()
NAMED_UNIT(*)
SI_UNIT(.MILLI.,.METRE.)
);
#9671=(
NAMED_UNIT(*)
PLANE_ANGLE_UNIT()
SI_UNIT($,.RADIAN.)
);
#9672=(
NAMED_UNIT(*)
SI_UNIT($,.STERADIAN.)
SOLID_ANGLE_UNIT()
);
#9682=SHAPE_DEFINITION_REPRESENTATION(#9694,#9720);
#9694=PRODUCT_DEFINITION_SHAPE('',$,#9733);
#9720=SHAPE_REPRESENTATION('',(#4326),#9665);
#9723=PRODUCT_DEFINITION_CONTEXT('part definition',#9761,'design');
#9733=PRODUCT_DEFINITION('2026-10-04-08-13-48-888','HANDWHEEL',#9745,#9723);
#9745=PRODUCT_DEFINITION_FORMATION('',$,#9772);
#9761=APPLICATION_CONTEXT(
'Core Data for Automotive Mechanical Design Process');
#9762=PRODUCT_CONTEXT('part definition',#9761,'mechanical');
#9772=PRODUCT('2026-10-04-08-13-48-888','HANDWHEEL','PART',(#9762));
#9775=PRESENTATION_STYLE_ASSIGNMENT((#9776));
#9776=SURFACE_STYLE_USAGE(.BOTH.,#9777);
#9777=SURFACE_SIDE_STYLE('',(#9778));
#9778=SURFACE_STYLE_FILL_AREA(#9779);
#9779=FILL_AREA_STYLE('Steel - Satin',(#9780));
#9780=FILL_AREA_STYLE_COLOUR('Steel - Satin',#9781);
#9781=COLOUR_RGB('Steel - Satin', 0.09019608, 0.27058824, 0.51372549);
ENDSEC;
END-ISO-10303-21;
